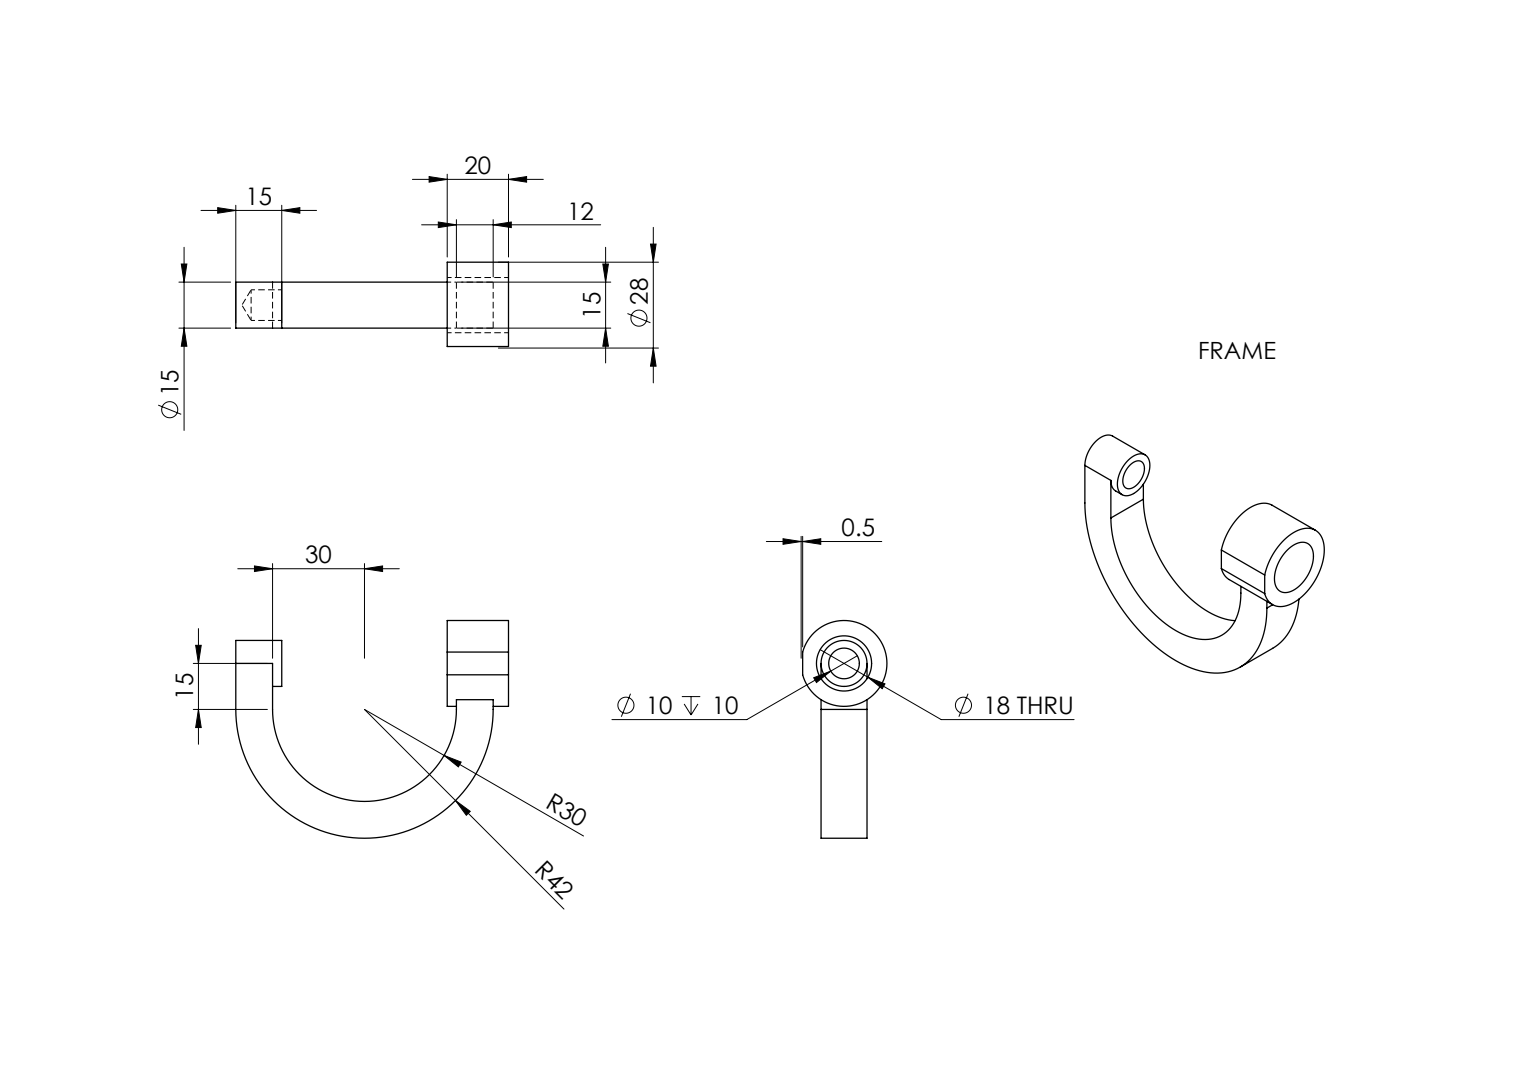
ISO-10303-21;
HEADER;
FILE_DESCRIPTION (('STEP AP214'),
    '1' );
FILE_NAME ('frame.step',
    '2026-10-22T12:35:56',
    ( '' ),
    ( '' ),
    'SwSTEP 2.0',
    'SolidWorks 2026',
    '' );
FILE_SCHEMA (( 'AUTOMOTIVE_DESIGN' ));
ENDSEC;

DATA;
#1=CARTESIAN_POINT ( 'NONE',  ( -30.00000000000000000, -8.316621552948000372E-15, 7.500000000000000000 ) ) ;
#2=ORIENTED_EDGE ( 'NONE', *, *, #1476, .F. ) ;
#4=DIRECTION ( 'NONE',  ( 0.000000000000000000, -1.000000000000000000, 0.000000000000000000 ) ) ;
#7=EDGE_CURVE ( 'NONE', #417, #1789, #1947, .T. ) ;
#12=VECTOR ( 'NONE', #2247, 1000.000000000000000 ) ;
#13=ORIENTED_EDGE ( 'NONE', *, *, #713, .T. ) ;
#15=CARTESIAN_POINT ( 'NONE',  ( 41.99999999999999289, -11.82159041753687845, 15.00000000000000000 ) ) ;
#16=CARTESIAN_POINT ( 'NONE',  ( 37.48326775981565362, -1.423407605072588344, 16.38680797912482134 ) ) ;
#23=CARTESIAN_POINT ( 'NONE',  ( -26.99999999999999645, -7.622732162557277534E-15, 7.500000000000000000 ) ) ;
#32=CIRCLE ( 'NONE', #2124, 4.999999999999998224 ) ;
#33=CARTESIAN_POINT ( 'NONE',  ( 30.00000000000000355, -15.00000000000000355, 15.00000000000000000 ) ) ;
#40=DIRECTION ( 'NONE',  ( 0.000000000000000000, 0.000000000000000000, -1.000000000000000000 ) ) ;
#47=DIRECTION ( 'NONE',  ( 0.5150380749100542666, 1.049727191138618572E-16, 0.8571673007021122226 ) ) ;
#51=EDGE_CURVE ( 'NONE', #357, #1877, #2331, .T. ) ;
#54=CARTESIAN_POINT ( 'NONE',  ( 35.50000000000001421, 0.09798730130381244630, 16.49999999999999645 ) ) ;
#56=VERTEX_POINT ( 'NONE', #623 ) ;
#57=ORIENTED_EDGE ( 'NONE', *, *, #1286, .T. ) ;
#60=DIRECTION ( 'NONE',  ( -2.478176394252581634E-16, 1.000000000000000000, 0.000000000000000000 ) ) ;
#63=COLOUR_RGB ( '',0.8941176470588234615, 0.8941176470588234615, 0.8941176470588234615 ) ;
#64=ORIENTED_EDGE ( 'NONE', *, *, #1192, .F. ) ;
#66=AXIS2_PLACEMENT_3D ( 'NONE', #1107, #1144, #2625 ) ;
#69=ORIENTED_EDGE ( 'NONE', *, *, #671, .F. ) ;
#71=CARTESIAN_POINT ( 'NONE',  ( 38.30162487582177278, 0.7519129166725618818, 16.46890859085320358 ) ) ;
#72=DIRECTION ( 'NONE',  ( -0.000000000000000000, -0.000000000000000000, 1.000000000000000000 ) ) ;
#73=CARTESIAN_POINT ( 'NONE',  ( 36.00776062886355078, -1.129166992945587866, 16.42915638304272363 ) ) ;
#76=EDGE_CURVE ( 'NONE', #916, #1503, #2106, .T. ) ;
#77=DIRECTION ( 'NONE',  ( 1.000000000000000000, 2.312964634635742957E-16, 0.000000000000000000 ) ) ;
#81=AXIS2_PLACEMENT_3D ( 'NONE', #778, #1048, #1778 ) ;
#86=DIRECTION ( 'NONE',  ( -2.312964634635742957E-16, 1.000000000000000000, 0.000000000000000000 ) ) ;
#87=VERTEX_POINT ( 'NONE', #874 ) ;
#96=ORIENTED_EDGE ( 'NONE', *, *, #1476, .T. ) ;
#97=ORIENTED_EDGE ( 'NONE', *, *, #671, .T. ) ;
#99=CARTESIAN_POINT ( 'NONE',  ( 37.00000000000000000, 1.474514954580286030E-14, 20.99999999999999645 ) ) ;
#102=AXIS2_PLACEMENT_3D ( 'NONE', #2450, #1198, #3216 ) ;
#107=CARTESIAN_POINT ( 'NONE',  ( 38.45998082922275785, -0.3957415549423216605, 16.49311123862704775 ) ) ;
#116=VECTOR ( 'NONE', #3173, 1000.000000000000000 ) ;
#118=DIRECTION ( 'NONE',  ( 0.000000000000000000, 0.000000000000000000, -1.000000000000000000 ) ) ;
#120=DIRECTION ( 'NONE',  ( 1.000000000000000000, 2.312964634635742957E-16, -0.000000000000000000 ) ) ;
#121=AXIS2_PLACEMENT_3D ( 'NONE', #2014, #774, #60 ) ;
#127=ADVANCED_FACE ( 'NONE', ( #378 ), #1155, .F. ) ;
#128=ADVANCED_FACE ( 'NONE', ( #911 ), #1859, .T. ) ;
#129=ORIENTED_EDGE ( 'NONE', *, *, #314, .F. ) ;
#134=CYLINDRICAL_SURFACE ( 'NONE', #2744, 14.00000000000000000 ) ;
#136=ORIENTED_EDGE ( 'NONE', *, *, #525, .F. ) ;
#147=EDGE_CURVE ( 'NONE', #1882, #2430, #639, .T. ) ;
#148=CYLINDRICAL_SURFACE ( 'NONE', #941, 7.500000000000000000 ) ;
#158=CARTESIAN_POINT ( 'NONE',  ( 41.99999999999999289, 6.449497959004948951E-15, 15.00000000000000000 ) ) ;
#163=VERTEX_POINT ( 'NONE', #411 ) ;
#167=DIRECTION ( 'NONE',  ( -0.000000000000000000, -0.000000000000000000, -1.000000000000000000 ) ) ;
#172=AXIS2_PLACEMENT_3D ( 'NONE', #834, #880, #1605 ) ;
#177=ORIENTED_EDGE ( 'NONE', *, *, #295, .F. ) ;
#190=DIRECTION ( 'NONE',  ( 1.000000000000000000, -0.000000000000000000, -0.000000000000000000 ) ) ;
#193=CIRCLE ( 'NONE', #2951, 14.00000000000000000 ) ;
#198=CYLINDRICAL_SURFACE ( 'NONE', #340, 1.499999999999994449 ) ;
#204=LINE ( 'NONE', #1443, #277 ) ;
#206=CONICAL_SURFACE ( 'NONE', #1038, 4.999999999999998224, 1.029744258676654312 ) ;
#210=ADVANCED_FACE ( 'NONE', ( #1707 ), #1221, .T. ) ;
#216=CARTESIAN_POINT ( 'NONE',  ( -41.99999999999999289, -6.449497959004950529E-15, 0.000000000000000000 ) ) ;
#217=DIRECTION ( 'NONE',  ( 0.000000000000000000, 0.000000000000000000, -1.000000000000000000 ) ) ;
#218=DIRECTION ( 'NONE',  ( 1.000000000000000000, 0.000000000000000000, 0.000000000000000000 ) ) ;
#224=AXIS2_PLACEMENT_3D ( 'NONE', #361, #2327, #86 ) ;
#226=AXIS2_PLACEMENT_3D ( 'NONE', #781, #362, #1550 ) ;
#227=DIRECTION ( 'NONE',  ( -1.000000000000000000, -2.312964634635742957E-16, 0.000000000000000000 ) ) ;
#231=ORIENTED_EDGE ( 'NONE', *, *, #2924, .F. ) ;
#232=EDGE_LOOP ( 'NONE', ( #1435, #2607, #784, #823 ) ) ;
#246=CIRCLE ( 'NONE', #2580, 14.00000000000000000 ) ;
#247=ORIENTED_EDGE ( 'NONE', *, *, #3182, .F. ) ;
#254=PRODUCT_DEFINITION ( 'UNKNOWN', '', #1654, #571 ) ;
#259=CARTESIAN_POINT ( 'NONE',  ( 27.00000000000000000, 6.704247063196759979E-15, 7.500000000000000000 ) ) ;
#266=DIRECTION ( 'NONE',  ( -2.478176394252581634E-16, 1.000000000000000000, 0.000000000000000000 ) ) ;
#273=EDGE_CURVE ( 'NONE', #3128, #417, #1689, .T. ) ;
#276=DIRECTION ( 'NONE',  ( 1.000000000000000000, 0.000000000000000000, 0.000000000000000000 ) ) ;
#277=VECTOR ( 'NONE', #2201, 1000.000000000000000 ) ;
#279=CARTESIAN_POINT ( 'NONE',  ( -41.99999999999999289, -1.109217911451089172E-14, 0.000000000000000000 ) ) ;
#282=CIRCLE ( 'NONE', #2213, 4.999999999999999112 ) ;
#287=CARTESIAN_POINT ( 'NONE',  ( 38.19805860116020568, -0.9234461779904078460, 16.45357685834587613 ) ) ;
#289=LINE ( 'NONE', #2050, #12 ) ;
#295=EDGE_CURVE ( 'NONE', #1128, #2739, #2239, .T. ) ;
#297=PLANE ( 'NONE',  #1247 ) ;
#299=ORIENTED_EDGE ( 'NONE', *, *, #397, .F. ) ;
#308=DIRECTION ( 'NONE',  ( -1.000000000000000000, -2.312964634635742957E-16, 0.000000000000000000 ) ) ;
#313=FACE_OUTER_BOUND ( 'NONE', #2374, .T. ) ;
#314=EDGE_CURVE ( 'NONE', #1882, #2739, #2737, .T. ) ;
#317=DIRECTION ( 'NONE',  ( -2.312964634635742957E-16, 1.000000000000000000, -0.000000000000000000 ) ) ;
#320=ORIENTED_EDGE ( 'NONE', *, *, #1335, .T. ) ;
#324=ORIENTED_EDGE ( 'NONE', *, *, #2185, .F. ) ;
#325=ADVANCED_FACE ( 'NONE', ( #447 ), #1432, .F. ) ;
#327=CARTESIAN_POINT ( 'NONE',  ( 38.49999999999999289, 1.474514954580286030E-14, 16.49999999999999289 ) ) ;
#329=EDGE_CURVE ( 'NONE', #2636, #2004, #2214, .T. ) ;
#333=CIRCLE ( 'NONE', #2770, 14.00000000000000000 ) ;
#335=CARTESIAN_POINT ( 'NONE',  ( -30.00000000000000000, -3.673940397442059178E-15, 0.000000000000000000 ) ) ;
#340=AXIS2_PLACEMENT_3D ( 'NONE', #664, #915, #276 ) ;
#341=AXIS2_PLACEMENT_3D ( 'NONE', #259, #1766, #1051 ) ;
#346=CYLINDRICAL_SURFACE ( 'NONE', #226, 14.00000000000000000 ) ;
#349=ORIENTED_EDGE ( 'NONE', *, *, #2340, .F. ) ;
#353=FACE_OUTER_BOUND ( 'NONE', #1646, .T. ) ;
#355=FACE_OUTER_BOUND ( 'NONE', #984, .T. ) ;
#357=VERTEX_POINT ( 'NONE', #15 ) ;
#361=CARTESIAN_POINT ( 'NONE',  ( 47.00000000000000000, 1.133017633246824530E-14, 7.500000000000000000 ) ) ;
#362=DIRECTION ( 'NONE',  ( 1.000000000000000000, 2.312964634635742957E-16, 0.000000000000000000 ) ) ;
#363=DIRECTION ( 'NONE',  ( -0.000000000000000000, -0.000000000000000000, -1.000000000000000000 ) ) ;
#366=CARTESIAN_POINT ( 'NONE',  ( 38.50000000000000000, -0.1985404316418107051, 16.49999999999999645 ) ) ;
#367=ORIENTED_EDGE ( 'NONE', *, *, #1335, .F. ) ;
#372=EDGE_CURVE ( 'NONE', #87, #2397, #1009, .T. ) ;
#378=FACE_OUTER_BOUND ( 'NONE', #1451, .T. ) ;
#382=ORIENTED_EDGE ( 'NONE', *, *, #1088, .F. ) ;
#386=AXIS2_PLACEMENT_3D ( 'NONE', #1799, #2316, #40 ) ;
#389=EDGE_LOOP ( 'NONE', ( #1124, #807, #247, #64 ) ) ;
#390=AXIS2_PLACEMENT_3D ( 'NONE', #3020, #1047, #980 ) ;
#392=VECTOR ( 'NONE', #317, 1000.000000000000000 ) ;
#393=DIRECTION ( 'NONE',  ( -1.000000000000000000, -2.312964634635742957E-16, 0.000000000000000000 ) ) ;
#397=EDGE_CURVE ( 'NONE', #1789, #2998, #1521, .T. ) ;
#410=VECTOR ( 'NONE', #420, 1000.000000000000000 ) ;
#411=CARTESIAN_POINT ( 'NONE',  ( 27.00000000000000000, 1.243235845170086479E-14, 16.49999999999999289 ) ) ;
#417=VERTEX_POINT ( 'NONE', #1239 ) ;
#420=DIRECTION ( 'NONE',  ( 1.000000000000000000, 2.312964634635742957E-16, 0.000000000000000000 ) ) ;
#424=VECTOR ( 'NONE', #2474, 1000.000000000000000 ) ;
#434=DIRECTION ( 'NONE',  ( -2.312964634635742957E-16, 1.000000000000000000, 0.000000000000000000 ) ) ;
#435=DIRECTION ( 'NONE',  ( 1.000000000000000000, 2.312964634635742957E-16, 0.000000000000000000 ) ) ;
#440=CARTESIAN_POINT ( 'NONE',  ( -41.99999999999999289, -15.00000000000000711, 15.00000000000000000 ) ) ;
#443=CLOSED_SHELL ( 'NONE', ( #3157, #127, #2028, #1449, #2628, #1324, #3219, #537, #1757, #1948, #128, #2460, #2730, #325, #210, #2684, #2552, #1070, #2797, #829, #2086, #2736, #3198, #1675, #3211 ) ) ;
#447=FACE_OUTER_BOUND ( 'NONE', #1253, .T. ) ;
#450=CYLINDRICAL_SURFACE ( 'NONE', #386, 8.999999999999994671 ) ;
#452=CARTESIAN_POINT ( 'NONE',  ( -26.99999999999999645, -7.622732162557277534E-15, 7.500000000000000000 ) ) ;
#464=ORIENTED_EDGE ( 'NONE', *, *, #1403, .T. ) ;
#469=DIRECTION ( 'NONE',  ( -0.000000000000000000, -0.000000000000000000, -1.000000000000000000 ) ) ;
#470=DIRECTION ( 'NONE',  ( 0.000000000000000000, 0.000000000000000000, -1.000000000000000000 ) ) ;
#485=PRODUCT_CONTEXT ( 'NONE', #2078, 'mechanical' ) ;
#491=( GEOMETRIC_REPRESENTATION_CONTEXT ( 3 ) GLOBAL_UNCERTAINTY_ASSIGNED_CONTEXT ( ( #2017 ) ) GLOBAL_UNIT_ASSIGNED_CONTEXT ( ( #605, #1315, #1563 ) ) REPRESENTATION_CONTEXT ( 'NONE', 'WORKASPACE' ) );
#505=FACE_BOUND ( 'NONE', #645, .T. ) ;
#508=CARTESIAN_POINT ( 'NONE',  ( 35.50982285435565444, 0.1975270956567308500, 16.49834805537327043 ) ) ;
#511=DIRECTION ( 'NONE',  ( 1.000000000000000000, 0.000000000000000000, 0.000000000000000000 ) ) ;
#514=SHAPE_REPRESENTATION ( 'frame', ( #2878 ), #491 ) ;
#515=CIRCLE ( 'NONE', #769, 14.00000000000000000 ) ;
#522=DIRECTION ( 'NONE',  ( -0.000000000000000000, -0.000000000000000000, 1.000000000000000000 ) ) ;
#525=EDGE_CURVE ( 'NONE', #974, #2998, #2583, .T. ) ;
#526=CARTESIAN_POINT ( 'NONE',  ( 37.92226537325436198, 1.198992358192679797, 16.42086068928975706 ) ) ;
#529=ORIENTED_EDGE ( 'NONE', *, *, #1753, .F. ) ;
#530=CIRCLE ( 'NONE', #1202, 8.999999999999989342 ) ;
#532=DIRECTION ( 'NONE',  ( 1.000000000000000000, 2.312964634635742957E-16, 0.000000000000000000 ) ) ;
#533=CARTESIAN_POINT ( 'NONE',  ( 37.99089481476345753, -1.130332597043731901, 16.42900728359812135 ) ) ;
#537=ADVANCED_FACE ( 'NONE', ( #579 ), #1568, .T. ) ;
#538=CARTESIAN_POINT ( 'NONE',  ( -26.99999999999999645, -7.622732162557277534E-15, 7.500000000000000000 ) ) ;
#542=SURFACE_STYLE_FILL_AREA ( #2023 ) ;
#553=CARTESIAN_POINT ( 'NONE',  ( 35.68903409116789760, -0.7546922429561464529, 16.47012649564899078 ) ) ;
#559=EDGE_CURVE ( 'NONE', #3128, #1393, #1428, .T. ) ;
#561=CARTESIAN_POINT ( 'NONE',  ( 35.50000000000000000, 1.243235838461289750E-14, 16.49999999999999289 ) ) ;
#564=ORIENTED_EDGE ( 'NONE', *, *, #1430, .T. ) ;
#571=PRODUCT_DEFINITION_CONTEXT ( 'detailed design', #2741, 'design' ) ;
#574=DIRECTION ( 'NONE',  ( 1.000000000000000000, 0.000000000000000000, 0.000000000000000000 ) ) ;
#575=EDGE_CURVE ( 'NONE', #2092, #576, #3015, .T. ) ;
#576=VERTEX_POINT ( 'NONE', #1290 ) ;
#579=FACE_OUTER_BOUND ( 'NONE', #389, .T. ) ;
#585=VERTEX_POINT ( 'NONE', #1541 ) ;
#586=CARTESIAN_POINT ( 'NONE',  ( -26.99999999999999645, -5.173438564262573782E-15, 12.49999999999999822 ) ) ;
#593=CARTESIAN_POINT ( 'NONE',  ( -30.00000000000000000, -3.673940397442059178E-15, 0.000000000000000000 ) ) ;
#596=ORIENTED_EDGE ( 'NONE', *, *, #1551, .F. ) ;
#598=EDGE_CURVE ( 'NONE', #1829, #1709, #1645, .T. ) ;
#599=VECTOR ( 'NONE', #47, 1000.000000000000000 ) ;
#600=AXIS2_PLACEMENT_3D ( 'NONE', #3063, #77, #3053 ) ;
#605=( LENGTH_UNIT ( ) NAMED_UNIT ( * ) SI_UNIT ( .MILLI., .METRE. ) );
#612=CARTESIAN_POINT ( 'NONE',  ( -26.99999999999999645, -5.785761963836251101E-15, 2.500000000000000444 ) ) ;
#613=AXIS2_PLACEMENT_3D ( 'NONE', #951, #1199, #470 ) ;
#623=CARTESIAN_POINT ( 'NONE',  ( -40.00430309513780003, -9.040569623688697978E-15, 7.500000000000000000 ) ) ;
#629=DIRECTION ( 'NONE',  ( -2.312964634635742957E-16, 1.000000000000000000, 0.000000000000000000 ) ) ;
#631=DIRECTION ( 'NONE',  ( -0.000000000000000000, -0.000000000000000000, -1.000000000000000000 ) ) ;
#639=LINE ( 'NONE', #1636, #1796 ) ;
#640=VERTEX_POINT ( 'NONE', #1514 ) ;
#645=EDGE_LOOP ( 'NONE', ( #2403, #3181 ) ) ;
#647=AXIS2_PLACEMENT_3D ( 'NONE', #686, #2975, #2223 ) ;
#650=CIRCLE ( 'NONE', #1368, 8.999999999999994671 ) ;
#654=AXIS2_PLACEMENT_3D ( 'NONE', #452, #2165, #917 ) ;
#657=EDGE_CURVE ( 'NONE', #1365, #640, #2412, .T. ) ;
#659=DIRECTION ( 'NONE',  ( 0.000000000000000000, 0.000000000000000000, -1.000000000000000000 ) ) ;
#662=DIRECTION ( 'NONE',  ( 1.000000000000000000, 2.312964634635742957E-16, 0.000000000000000000 ) ) ;
#664=CARTESIAN_POINT ( 'NONE',  ( 37.00000000000000000, 1.474514954580286030E-14, 20.99999999999999645 ) ) ;
#668=LINE ( 'NONE', #730, #1764 ) ;
#671=EDGE_CURVE ( 'NONE', #1489, #1964, #2710, .T. ) ;
#673=VECTOR ( 'NONE', #1742, 1000.000000000000000 ) ;
#682=CARTESIAN_POINT ( 'NONE',  ( 30.00000000000000355, -11.82159041753688200, 15.00000000000000000 ) ) ;
#686=CARTESIAN_POINT ( 'NONE',  ( 3.469446951953614189E-15, -15.00000000000000355, 15.00000000000000000 ) ) ;
#687=ORIENTED_EDGE ( 'NONE', *, *, #1176, .F. ) ;
#690=EDGE_LOOP ( 'NONE', ( #13, #3111, #3143, #1378, #349, #2589 ) ) ;
#693=CARTESIAN_POINT ( 'NONE',  ( -37.00000000000000000, -5.785761963836251101E-15, 2.500000000000001332 ) ) ;
#695=CARTESIAN_POINT ( 'NONE',  ( -29.99999999999999645, -15.00000000000000355, 15.00000000000000000 ) ) ;
#698=FACE_OUTER_BOUND ( 'NONE', #2603, .T. ) ;
#702=VECTOR ( 'NONE', #227, 1000.000000000000000 ) ;
#710=DIRECTION ( 'NONE',  ( 1.000000000000000000, -0.000000000000000000, -0.000000000000000000 ) ) ;
#713=EDGE_CURVE ( 'NONE', #1393, #3128, #2675, .T. ) ;
#727=DIRECTION ( 'NONE',  ( 0.000000000000000000, 1.000000000000000000, 0.000000000000000000 ) ) ;
#729=FACE_OUTER_BOUND ( 'NONE', #989, .T. ) ;
#730=CARTESIAN_POINT ( 'NONE',  ( 30.00000000000000355, -15.00000000000000355, 15.00000000000000000 ) ) ;
#732=DIRECTION ( 'NONE',  ( 1.000000000000000000, 2.312964634635742957E-16, 0.000000000000000000 ) ) ;
#736=CARTESIAN_POINT ( 'NONE',  ( 41.99999999999999289, -11.82159041753688022, 0.000000000000000000 ) ) ;
#741=FACE_OUTER_BOUND ( 'NONE', #2868, .T. ) ;
#746=VECTOR ( 'NONE', #732, 1000.000000000000000 ) ;
#750=DIRECTION ( 'NONE',  ( -0.000000000000000000, -0.000000000000000000, -1.000000000000000000 ) ) ;
#756=CARTESIAN_POINT ( 'NONE',  ( -37.00000000000000000, -5.173438564262574571E-15, 12.49999999999999645 ) ) ;
#762=DIRECTION ( 'NONE',  ( 1.000000000000000000, 0.000000000000000000, 0.000000000000000000 ) ) ;
#769=AXIS2_PLACEMENT_3D ( 'NONE', #3204, #435, #2416 ) ;
#772=EDGE_CURVE ( 'NONE', #1678, #1779, #333, .T. ) ;
#774=DIRECTION ( 'NONE',  ( 1.000000000000000000, 2.312964634635742957E-16, -0.000000000000000000 ) ) ;
#776=( LENGTH_UNIT ( ) NAMED_UNIT ( * ) SI_UNIT ( .MILLI., .METRE. ) );
#777=UNCERTAINTY_MEASURE_WITH_UNIT (LENGTH_MEASURE( 1.000000000000000082E-05 ), #1533, 'distance_accuracy_value', 'NONE');
#778=CARTESIAN_POINT ( 'NONE',  ( -41.99999999999999289, -1.109217911451089172E-14, 7.500000000000000000 ) ) ;
#779=VERTEX_POINT ( 'NONE', #586 ) ;
#781=CARTESIAN_POINT ( 'NONE',  ( 27.00000000000000000, 6.704247063196759979E-15, 7.500000000000000000 ) ) ;
#782=CARTESIAN_POINT ( 'NONE',  ( -26.99999999999999645, -5.785761963836251101E-15, 7.500000000000000000 ) ) ;
#784=ORIENTED_EDGE ( 'NONE', *, *, #2418, .T. ) ;
#790=AXIS2_PLACEMENT_3D ( 'NONE', #2216, #1953, #2198 ) ;
#792=LINE ( 'NONE', #2780, #2329 ) ;
#796=CARTESIAN_POINT ( 'NONE',  ( 35.54829862735515889, 0.3901384415568778796, 16.49205630963118807 ) ) ;
#801=( GEOMETRIC_REPRESENTATION_CONTEXT ( 3 ) GLOBAL_UNCERTAINTY_ASSIGNED_CONTEXT ( ( #1879 ) ) GLOBAL_UNIT_ASSIGNED_CONTEXT ( ( #776, #1509, #3040 ) ) REPRESENTATION_CONTEXT ( 'NONE', 'WORKASPACE' ) );
#802=ORIENTED_EDGE ( 'NONE', *, *, #575, .T. ) ;
#804=DIRECTION ( 'NONE',  ( 0.000000000000000000, -1.000000000000000000, 0.000000000000000000 ) ) ;
#807=ORIENTED_EDGE ( 'NONE', *, *, #1490, .T. ) ;
#818=LINE ( 'NONE', #756, #599 ) ;
#823=ORIENTED_EDGE ( 'NONE', *, *, #2248, .T. ) ;
#825=CARTESIAN_POINT ( 'NONE',  ( 35.80758137781341333, 0.9152444266664423456, 16.45371270176149991 ) ) ;
#826=FILL_AREA_STYLE_COLOUR ( '', #63 ) ;
#829=ADVANCED_FACE ( 'NONE', ( #1330, #2376 ), #1614, .T. ) ;
#833=ORIENTED_EDGE ( 'NONE', *, *, #2536, .F. ) ;
#834=CARTESIAN_POINT ( 'NONE',  ( 27.00000000000000000, 1.133017633246824530E-14, 7.500000000000000000 ) ) ;
#835=DIRECTION ( 'NONE',  ( 1.000000000000000000, 2.312964634635742957E-16, 0.000000000000000000 ) ) ;
#837=DIRECTION ( 'NONE',  ( -0.000000000000000000, -0.000000000000000000, -1.000000000000000000 ) ) ;
#839=EDGE_CURVE ( 'NONE', #1877, #916, #3032, .T. ) ;
#840=ORIENTED_EDGE ( 'NONE', *, *, #1067, .T. ) ;
#846=CARTESIAN_POINT ( 'NONE',  ( -29.99999999999999645, -15.00000000000000355, 15.00000000000000000 ) ) ;
#859=ORIENTED_EDGE ( 'NONE', *, *, #1403, .F. ) ;
#864=CIRCLE ( 'NONE', #81, 7.500000000000000000 ) ;
#869=VECTOR ( 'NONE', #662, 1000.000000000000000 ) ;
#871=FACE_OUTER_BOUND ( 'NONE', #3146, .T. ) ;
#874=CARTESIAN_POINT ( 'NONE',  ( 47.00000000000000000, -13.99999999999998757, 7.500000000000001776 ) ) ;
#877=VERTEX_POINT ( 'NONE', #2663 ) ;
#880=DIRECTION ( 'NONE',  ( 1.000000000000000000, 2.312964634635742957E-16, 0.000000000000000000 ) ) ;
#883=CARTESIAN_POINT ( 'NONE',  ( 47.00000000000000000, 1.133017633246824530E-14, 7.500000000000000000 ) ) ;
#893=EDGE_CURVE ( 'NONE', #2713, #2821, #204, .T. ) ;
#895=ORIENTED_EDGE ( 'NONE', *, *, #314, .T. ) ;
#900=AXIS2_PLACEMENT_3D ( 'NONE', #2362, #363, #3105 ) ;
#907=PRODUCT_DEFINITION_SHAPE ( 'NONE', 'NONE',  #254 ) ;
#911=FACE_OUTER_BOUND ( 'NONE', #2074, .T. ) ;
#915=DIRECTION ( 'NONE',  ( -0.000000000000000000, -0.000000000000000000, 1.000000000000000000 ) ) ;
#916=VERTEX_POINT ( 'NONE', #440 ) ;
#917=DIRECTION ( 'NONE',  ( 0.000000000000000000, -1.000000000000000000, 0.000000000000000000 ) ) ;
#918=CARTESIAN_POINT ( 'NONE',  ( -26.99999999999999645, -5.785761963836251101E-15, 7.500000000000000000 ) ) ;
#924=CARTESIAN_POINT ( 'NONE',  ( 27.00000000000000355, -11.82159041753688200, 15.00000000000000000 ) ) ;
#930=CARTESIAN_POINT ( 'NONE',  ( 52.00000000000000711, 3.708099243547853252, 20.99999999999999645 ) ) ;
#931=EDGE_CURVE ( 'NONE', #1570, #585, #2261, .T. ) ;
#933=ORIENTED_EDGE ( 'NONE', *, *, #2759, .F. ) ;
#941=AXIS2_PLACEMENT_3D ( 'NONE', #1146, #2146, #3131 ) ;
#943=EDGE_CURVE ( 'NONE', #2713, #357, #3155, .T. ) ;
#951=CARTESIAN_POINT ( 'NONE',  ( -37.00000000000000000, -5.785761963836251101E-15, 7.500000000000000000 ) ) ;
#960=PLANE ( 'NONE',  #1825 ) ;
#962=ORIENTED_EDGE ( 'NONE', *, *, #893, .T. ) ;
#966=FACE_OUTER_BOUND ( 'NONE', #1512, .T. ) ;
#973=CARTESIAN_POINT ( 'NONE',  ( 41.99999999999999289, -15.00000000000000355, 15.00000000000000000 ) ) ;
#974=VERTEX_POINT ( 'NONE', #1187 ) ;
#978=CARTESIAN_POINT ( 'NONE',  ( -30.00000000000000000, -7.500000000000007994, 7.500000000000000000 ) ) ;
#980=DIRECTION ( 'NONE',  ( 0.000000000000000000, 0.000000000000000000, -1.000000000000000000 ) ) ;
#984=EDGE_LOOP ( 'NONE', ( #2241, #2447, #2019, #1978, #3024, #2576, #596, #895 ) ) ;
#989=EDGE_LOOP ( 'NONE', ( #2526, #57, #564, #96, #3116, #3195, #136, #1328 ) ) ;
#992=CARTESIAN_POINT ( 'NONE',  ( 36.60604563826976943, -1.460666791800804498, 16.38100777177576362 ) ) ;
#1002=CARTESIAN_POINT ( 'NONE',  ( 35.86950496355626683, 0.9908260551213666778, 16.44556929574713777 ) ) ;
#1005=DIRECTION ( 'NONE',  ( -0.000000000000000000, -0.000000000000000000, 1.000000000000000000 ) ) ;
#1007=LINE ( 'NONE', #2488, #424 ) ;
#1009=CIRCLE ( 'NONE', #2315, 14.00000000000000000 ) ;
#1012=ORIENTED_EDGE ( 'NONE', *, *, #772, .T. ) ;
#1021=AXIS2_PLACEMENT_3D ( 'NONE', #1457, #2451, #218 ) ;
#1031=CONICAL_SURFACE ( 'NONE', #613, 4.999999999999998224, 1.029744258676654312 ) ;
#1033=ORIENTED_EDGE ( 'NONE', *, *, #2418, .F. ) ;
#1036=PRESENTATION_STYLE_ASSIGNMENT (( #1283 ) ) ;
#1038=AXIS2_PLACEMENT_3D ( 'NONE', #2152, #1475, #2436 ) ;
#1040=CARTESIAN_POINT ( 'NONE',  ( -26.99999999999999645, -7.622732162557277534E-15, 7.500000000000000000 ) ) ;
#1041=CARTESIAN_POINT ( 'NONE',  ( 36.08479696852054985, -1.192462354422064497, 16.42082098627955844 ) ) ;
#1046=AXIS2_PLACEMENT_3D ( 'NONE', #2529, #2745, #266 ) ;
#1047=DIRECTION ( 'NONE',  ( 1.000000000000000000, -0.000000000000000000, -0.000000000000000000 ) ) ;
#1048=DIRECTION ( 'NONE',  ( -1.000000000000000000, -2.312964634635742957E-16, 0.000000000000000000 ) ) ;
#1050=ADVANCED_BREP_SHAPE_REPRESENTATION ( '', ( #2136, #2878 ), #491 ) ;
#1051=DIRECTION ( 'NONE',  ( -2.478176394252581634E-16, 1.000000000000000000, 0.000000000000000000 ) ) ;
#1052=FACE_OUTER_BOUND ( 'NONE', #1325, .T. ) ;
#1055=DIRECTION ( 'NONE',  ( -1.000000000000000000, -2.312964634635742957E-16, 0.000000000000000000 ) ) ;
#1056=ORIENTED_EDGE ( 'NONE', *, *, #1551, .T. ) ;
#1058=ORIENTED_EDGE ( 'NONE', *, *, #76, .F. ) ;
#1060=AXIS2_PLACEMENT_3D ( 'NONE', #1040, #1830, #804 ) ;
#1067=EDGE_CURVE ( 'NONE', #2004, #2636, #3079, .T. ) ;
#1068=DIRECTION ( 'NONE',  ( 0.000000000000000000, 1.000000000000000000, 0.000000000000000000 ) ) ;
#1069=ORIENTED_EDGE ( 'NONE', *, *, #1430, .F. ) ;
#1070=ADVANCED_FACE ( 'NONE', ( #505, #1762 ), #1495, .F. ) ;
#1071=CARTESIAN_POINT ( 'NONE',  ( 36.80294994545206322, 1.490236770648136089, 16.37578575999040353 ) ) ;
#1072=ORIENTED_EDGE ( 'NONE', *, *, #7, .T. ) ;
#1077=LINE ( 'NONE', #612, #2159 ) ;
#1079=EDGE_LOOP ( 'NONE', ( #933, #177, #3058, #1169 ) ) ;
#1080=EDGE_CURVE ( 'NONE', #2998, #1599, #2718, .T. ) ;
#1082=( NAMED_UNIT ( * ) PLANE_ANGLE_UNIT ( ) SI_UNIT ( $, .RADIAN. ) );
#1087=CARTESIAN_POINT ( 'NONE',  ( 30.00000000000000000, 3.673940397442057600E-15, 0.000000000000000000 ) ) ;
#1088=EDGE_CURVE ( 'NONE', #1709, #1829, #32, .T. ) ;
#1092=EDGE_CURVE ( 'NONE', #3031, #417, #864, .T. ) ;
#1097=DIRECTION ( 'NONE',  ( 1.000000000000000000, 0.000000000000000000, 0.000000000000000000 ) ) ;
#1105=VECTOR ( 'NONE', #1744, 1000.000000000000000 ) ;
#1106=ORIENTED_EDGE ( 'NONE', *, *, #1172, .F. ) ;
#1107=CARTESIAN_POINT ( 'NONE',  ( 3.469446951953614189E-15, -15.00000000000000355, 15.00000000000000000 ) ) ;
#1110=CARTESIAN_POINT ( 'NONE',  ( 47.00000000000000000, 14.00000000000001243, 7.500000000000000000 ) ) ;
#1124=ORIENTED_EDGE ( 'NONE', *, *, #1408, .F. ) ;
#1127=EDGE_CURVE ( 'NONE', #3031, #1482, #792, .T. ) ;
#1128=VERTEX_POINT ( 'NONE', #2544 ) ;
#1132=VECTOR ( 'NONE', #1607, 1000.000000000000000 ) ;
#1133=CARTESIAN_POINT ( 'NONE',  ( 27.00000000000000000, 6.704247063196759979E-15, 7.500000000000000000 ) ) ;
#1134=VERTEX_POINT ( 'NONE', #2295 ) ;
#1141=ORIENTED_EDGE ( 'NONE', *, *, #76, .T. ) ;
#1144=DIRECTION ( 'NONE',  ( -0.000000000000000000, -0.000000000000000000, -1.000000000000000000 ) ) ;
#1146=CARTESIAN_POINT ( 'NONE',  ( -26.99999999999999645, -7.622732162557277534E-15, 7.500000000000000000 ) ) ;
#1148=CARTESIAN_POINT ( 'NONE',  ( 27.00000000000000355, -13.99999999999999467, 7.500000000000001776 ) ) ;
#1155=CYLINDRICAL_SURFACE ( 'NONE', #1262, 8.999999999999994671 ) ;
#1165=CARTESIAN_POINT ( 'NONE',  ( 26.99999999999999645, 14.00000000000000711, 7.500000000000000000 ) ) ;
#1169=ORIENTED_EDGE ( 'NONE', *, *, #657, .F. ) ;
#1171=DIRECTION ( 'NONE',  ( 0.000000000000000000, 0.000000000000000000, -1.000000000000000000 ) ) ;
#1172=EDGE_CURVE ( 'NONE', #1877, #877, #3057, .T. ) ;
#1176=EDGE_CURVE ( 'NONE', #1134, #1570, #1853, .T. ) ;
#1187=CARTESIAN_POINT ( 'NONE',  ( -29.99999999999999645, -15.00000000000000355, 0.000000000000000000 ) ) ;
#1192=EDGE_CURVE ( 'NONE', #2397, #2430, #193, .T. ) ;
#1195=DIRECTION ( 'NONE',  ( -1.000000000000000000, -2.312964634635743450E-16, -0.000000000000000000 ) ) ;
#1198=DIRECTION ( 'NONE',  ( 1.000000000000000000, 2.312964634635742957E-16, 0.000000000000000000 ) ) ;
#1199=DIRECTION ( 'NONE',  ( 1.000000000000000000, -0.000000000000000000, -0.000000000000000000 ) ) ;
#1201=CARTESIAN_POINT ( 'NONE',  ( 47.00000000000000000, 1.133017633246824530E-14, 7.500000000000000000 ) ) ;
#1202=AXIS2_PLACEMENT_3D ( 'NONE', #1630, #2958, #1171 ) ;
#1212=CARTESIAN_POINT ( 'NONE',  ( -30.00000000000000000, -8.316621552948000372E-15, 15.00000000000000000 ) ) ;
#1221=PLANE ( 'NONE',  #647 ) ;
#1225=ORIENTED_EDGE ( 'NONE', *, *, #2062, .T. ) ;
#1229=LINE ( 'NONE', #2968, #1309 ) ;
#1233=VECTOR ( 'NONE', #2894, 1000.000000000000000 ) ;
#1236=CARTESIAN_POINT ( 'NONE',  ( 3.469446951953614189E-15, -15.00000000000000355, 0.000000000000000000 ) ) ;
#1237=ORIENTED_EDGE ( 'NONE', *, *, #295, .T. ) ;
#1239=CARTESIAN_POINT ( 'NONE',  ( -41.99999999999999289, 7.499999999999988454, 7.500000000000000888 ) ) ;
#1247=AXIS2_PLACEMENT_3D ( 'NONE', #3011, #1055, #2024 ) ;
#1248=CARTESIAN_POINT ( 'NONE',  ( 38.12949724085409997, 0.9918543271721460552, 16.44544909559322932 ) ) ;
#1249=CARTESIAN_POINT ( 'NONE',  ( -26.99999999999999645, 7.499999999999992006, 7.500000000000000888 ) ) ;
#1253=EDGE_LOOP ( 'NONE', ( #1918, #1934, #2174, #320 ) ) ;
#1254=DIRECTION ( 'NONE',  ( 1.000000000000000000, 2.312964634635743450E-16, 0.000000000000000000 ) ) ;
#1255=CARTESIAN_POINT ( 'NONE',  ( 36.80088933932602657, -1.499879510127380522, 16.37414004115126431 ) ) ;
#1258=AXIS2_PLACEMENT_3D ( 'NONE', #2990, #522, #762 ) ;
#1260=CARTESIAN_POINT ( 'NONE',  ( -37.00000000000000000, -5.785761963836251101E-15, 7.500000000000000000 ) ) ;
#1262=AXIS2_PLACEMENT_3D ( 'NONE', #2618, #2901, #659 ) ;
#1271=AXIS2_PLACEMENT_3D ( 'NONE', #23, #2252, #4 ) ;
#1277=CARTESIAN_POINT ( 'NONE',  ( -26.99999999999999645, -5.785761963836251101E-15, 7.500000000000000000 ) ) ;
#1280=ORIENTED_EDGE ( 'NONE', *, *, #329, .F. ) ;
#1283=SURFACE_STYLE_USAGE ( .BOTH. , #1597 ) ;
#1286=EDGE_CURVE ( 'NONE', #2092, #1779, #1374, .T. ) ;
#1290=CARTESIAN_POINT ( 'NONE',  ( 30.00000000000000355, -15.00000000000000355, 0.000000000000000000 ) ) ;
#1292=CARTESIAN_POINT ( 'NONE',  ( -26.99999999999999645, -5.173438564262573782E-15, 12.49999999999999822 ) ) ;
#1293=EDGE_LOOP ( 'NONE', ( #2363, #69, #2551, #840 ) ) ;
#1294=DIRECTION ( 'NONE',  ( 0.000000000000000000, 0.000000000000000000, -1.000000000000000000 ) ) ;
#1295=DIRECTION ( 'NONE',  ( 1.000000000000000000, 2.312964634635743450E-16, 0.000000000000000000 ) ) ;
#1303=EDGE_CURVE ( 'NONE', #2965, #1482, #1593, .T. ) ;
#1309=VECTOR ( 'NONE', #1439, 1000.000000000000000 ) ;
#1314=CARTESIAN_POINT ( 'NONE',  ( 37.39427925860091051, 1.460378464396937304, 16.38104908776753277 ) ) ;
#1315=( NAMED_UNIT ( * ) PLANE_ANGLE_UNIT ( ) SI_UNIT ( $, .RADIAN. ) );
#1324=ADVANCED_FACE ( 'NONE', ( #355 ), #134, .T. ) ;
#1325=EDGE_LOOP ( 'NONE', ( #859, #2531, #1528, #2705, #1558, #97 ) ) ;
#1326=DIRECTION ( 'NONE',  ( -1.000000000000000000, -2.312964634635742957E-16, 0.000000000000000000 ) ) ;
#1328=ORIENTED_EDGE ( 'NONE', *, *, #1821, .F. ) ;
#1330=FACE_OUTER_BOUND ( 'NONE', #2812, .T. ) ;
#1335=EDGE_CURVE ( 'NONE', #2821, #576, #668, .T. ) ;
#1343=ORIENTED_EDGE ( 'NONE', *, *, #1408, .T. ) ;
#1348=DIRECTION ( 'NONE',  ( -2.312964634635742957E-16, 1.000000000000000000, 0.000000000000000000 ) ) ;
#1351=CARTESIAN_POINT ( 'NONE',  ( 38.49999999999999289, 1.474514954580286030E-14, 16.49999999999999289 ) ) ;
#1357=ORIENTED_EDGE ( 'NONE', *, *, #2924, .T. ) ;
#1358=ORIENTED_EDGE ( 'NONE', *, *, #1080, .T. ) ;
#1359=DIRECTION ( 'NONE',  ( -2.312964634635742957E-16, 1.000000000000000000, 0.000000000000000000 ) ) ;
#1360=CARTESIAN_POINT ( 'NONE',  ( 41.99999999999999289, 1.017369401515037180E-14, 7.500000000000000000 ) ) ;
#1365=VERTEX_POINT ( 'NONE', #1148 ) ;
#1368=AXIS2_PLACEMENT_3D ( 'NONE', #1909, #2016, #2777 ) ;
#1374=LINE ( 'NONE', #2067, #2691 ) ;
#1378=ORIENTED_EDGE ( 'NONE', *, *, #1127, .T. ) ;
#1379=CARTESIAN_POINT ( 'NONE',  ( 35.50000000000000000, 1.243235838461289750E-14, 16.49999999999999289 ) ) ;
#1389=ORIENTED_EDGE ( 'NONE', *, *, #2656, .F. ) ;
#1393=VERTEX_POINT ( 'NONE', #2927 ) ;
#1401=LINE ( 'NONE', #3147, #2161 ) ;
#1403=EDGE_CURVE ( 'NONE', #163, #1964, #2183, .T. ) ;
#1405=CIRCLE ( 'NONE', #2651, 30.00000000000000000 ) ;
#1408=EDGE_CURVE ( 'NONE', #640, #2397, #2167, .T. ) ;
#1410=STYLED_ITEM('',(#3236),#2136);
#1411=ORIENTED_EDGE ( 'NONE', *, *, #1303, .F. ) ;
#1428=CIRCLE ( 'NONE', #1060, 7.500000000000000000 ) ;
#1430=EDGE_CURVE ( 'NONE', #1779, #877, #1715, .T. ) ;
#1432=CYLINDRICAL_SURFACE ( 'NONE', #2465, 30.00000000000000000 ) ;
#1434=DIRECTION ( 'NONE',  ( -1.000000000000000000, 0.000000000000000000, -0.000000000000000000 ) ) ;
#1435=ORIENTED_EDGE ( 'NONE', *, *, #1508, .F. ) ;
#1436=LINE ( 'NONE', #1693, #2002 ) ;
#1439=DIRECTION ( 'NONE',  ( -2.312964634635742957E-16, 1.000000000000000000, 0.000000000000000000 ) ) ;
#1440=CARTESIAN_POINT ( 'NONE',  ( 47.00000000000000000, 1.243235845170086321E-14, 16.49999999999999289 ) ) ;
#1443=CARTESIAN_POINT ( 'NONE',  ( 30.00000000000000000, 3.673940397442057600E-15, 15.00000000000000000 ) ) ;
#1449=ADVANCED_FACE ( 'NONE', ( #966 ), #1031, .F. ) ;
#1451=EDGE_LOOP ( 'NONE', ( #2053, #464, #1357, #2567, #2755, #687 ) ) ;
#1457=CARTESIAN_POINT ( 'NONE',  ( 3.469446951953614189E-15, -15.00000000000000355, 0.000000000000000000 ) ) ;
#1467=EDGE_LOOP ( 'NONE', ( #3062, #1889 ) ) ;
#1469=CARTESIAN_POINT ( 'NONE',  ( 41.99999999999999289, 1.017369401515037180E-14, 7.500000000000000000 ) ) ;
#1471=FACE_OUTER_BOUND ( 'NONE', #1079, .T. ) ;
#1475=DIRECTION ( 'NONE',  ( 1.000000000000000000, -0.000000000000000000, -0.000000000000000000 ) ) ;
#1476=EDGE_CURVE ( 'NONE', #877, #1503, #2429, .T. ) ;
#1481=AXIS2_PLACEMENT_3D ( 'NONE', #3076, #1846, #2772 ) ;
#1482=VERTEX_POINT ( 'NONE', #1212 ) ;
#1489=VERTEX_POINT ( 'NONE', #2957 ) ;
#1490=EDGE_CURVE ( 'NONE', #640, #1128, #515, .T. ) ;
#1494=DIRECTION ( 'NONE',  ( 1.000000000000000000, -0.000000000000000000, -0.000000000000000000 ) ) ;
#1495=PLANE ( 'NONE',  #2507 ) ;
#1497=ORIENTED_EDGE ( 'NONE', *, *, #2340, .T. ) ;
#1503=VERTEX_POINT ( 'NONE', #1729 ) ;
#1508=EDGE_CURVE ( 'NONE', #1709, #779, #1543, .T. ) ;
#1509=( NAMED_UNIT ( * ) PLANE_ANGLE_UNIT ( ) SI_UNIT ( $, .RADIAN. ) );
#1511=DIRECTION ( 'NONE',  ( -1.000000000000000000, -2.312964634635742957E-16, 0.000000000000000000 ) ) ;
#1512=EDGE_LOOP ( 'NONE', ( #833, #1770, #1669 ) ) ;
#1514=CARTESIAN_POINT ( 'NONE',  ( 26.99999999999999645, 14.00000000000000711, 7.500000000000000000 ) ) ;
#1521=LINE ( 'NONE', #216, #3141 ) ;
#1528=ORIENTED_EDGE ( 'NONE', *, *, #1176, .T. ) ;
#1532=CARTESIAN_POINT ( 'NONE',  ( 36.51683924005257609, 1.423460261948054750, 16.38679996801885252 ) ) ;
#1533=( LENGTH_UNIT ( ) NAMED_UNIT ( * ) SI_UNIT ( .MILLI., .METRE. ) );
#1534=DIRECTION ( 'NONE',  ( 1.000000000000000000, -0.000000000000000000, -0.000000000000000000 ) ) ;
#1538=ORIENTED_EDGE ( 'NONE', *, *, #839, .F. ) ;
#1541=CARTESIAN_POINT ( 'NONE',  ( 47.00000000000000000, 1.243235845170086321E-14, 16.49999999999998579 ) ) ;
#1542=CARTESIAN_POINT ( 'NONE',  ( 36.24736826332972583, -1.301195037071565030, 16.40561087244777738 ) ) ;
#1543=LINE ( 'NONE', #1292, #673 ) ;
#1548=ORIENTED_EDGE ( 'NONE', *, *, #2033, .F. ) ;
#1549=CARTESIAN_POINT ( 'NONE',  ( 38.19275052663392245, 0.9148478194932688767, 16.45375607287287423 ) ) ;
#1550=DIRECTION ( 'NONE',  ( -2.478176394252581634E-16, 1.000000000000000000, 0.000000000000000000 ) ) ;
#1551=EDGE_CURVE ( 'NONE', #1882, #87, #246, .T. ) ;
#1554=ORIENTED_EDGE ( 'NONE', *, *, #329, .T. ) ;
#1558=ORIENTED_EDGE ( 'NONE', *, *, #3166, .F. ) ;
#1560=DIRECTION ( 'NONE',  ( 0.000000000000000000, -1.000000000000000000, 0.000000000000000000 ) ) ;
#1561=VERTEX_POINT ( 'NONE', #3017 ) ;
#1563=( NAMED_UNIT ( * ) SI_UNIT ( $, .STERADIAN. ) SOLID_ANGLE_UNIT ( ) );
#1567=ORIENTED_EDGE ( 'NONE', *, *, #1127, .F. ) ;
#1568=CYLINDRICAL_SURFACE ( 'NONE', #600, 14.00000000000000000 ) ;
#1570=VERTEX_POINT ( 'NONE', #1997 ) ;
#1572=CARTESIAN_POINT ( 'NONE',  ( -30.00000000000000000, -8.316621552948000372E-15, 7.500000000000000000 ) ) ;
#1593=LINE ( 'NONE', #2323, #3059 ) ;
#1597=SURFACE_SIDE_STYLE ('',( #542 ) ) ;
#1599=VERTEX_POINT ( 'NONE', #978 ) ;
#1602=AXIS2_PLACEMENT_3D ( 'NONE', #930, #2381, #1434 ) ;
#1605=DIRECTION ( 'NONE',  ( -3.854941057726240069E-16, 1.000000000000000000, 0.000000000000000000 ) ) ;
#1607=DIRECTION ( 'NONE',  ( 1.000000000000000000, -0.000000000000000000, -0.000000000000000000 ) ) ;
#1614=PLANE ( 'NONE',  #224 ) ;
#1624=CARTESIAN_POINT ( 'NONE',  ( 47.00000000000000000, 3.708099243547851920, 20.99999999999999645 ) ) ;
#1627=CIRCLE ( 'NONE', #1046, 14.00000000000000000 ) ;
#1629=EDGE_LOOP ( 'NONE', ( #231, #1908, #1554, #1673 ) ) ;
#1630=CARTESIAN_POINT ( 'NONE',  ( 47.00000000000000000, 1.133017633246824530E-14, 7.500000000000000000 ) ) ;
#1631=DIRECTION ( 'NONE',  ( 0.000000000000000000, 1.000000000000000000, 0.000000000000000000 ) ) ;
#1636=CARTESIAN_POINT ( 'NONE',  ( 47.00000000000000000, 1.133017633246824530E-14, 20.99999999999999645 ) ) ;
#1639=VECTOR ( 'NONE', #1876, 1000.000000000000000 ) ;
#1640=AXIS2_PLACEMENT_3D ( 'NONE', #99, #72, #574 ) ;
#1641=AXIS2_PLACEMENT_3D ( 'NONE', #1572, #1326, #2822 ) ;
#1645=CIRCLE ( 'NONE', #1481, 4.999999999999998224 ) ;
#1646=EDGE_LOOP ( 'NONE', ( #1389, #3044, #1676, #1069, #2280 ) ) ;
#1654=PRODUCT_DEFINITION_FORMATION_WITH_SPECIFIED_SOURCE ( 'ANY', '', #2716, .NOT_KNOWN. ) ;
#1660=FACE_BOUND ( 'NONE', #1725, .T. ) ;
#1662=ORIENTED_EDGE ( 'NONE', *, *, #2188, .T. ) ;
#1665=ORIENTED_EDGE ( 'NONE', *, *, #372, .F. ) ;
#1669=ORIENTED_EDGE ( 'NONE', *, *, #1088, .T. ) ;
#1673=ORIENTED_EDGE ( 'NONE', *, *, #1793, .F. ) ;
#1675=ADVANCED_FACE ( 'NONE', ( #1660, #3162 ), #2669, .F. ) ;
#1676=ORIENTED_EDGE ( 'NONE', *, *, #1172, .T. ) ;
#1678=VERTEX_POINT ( 'NONE', #1880 ) ;
#1679=CARTESIAN_POINT ( 'NONE',  ( 35.50000000000000711, 1.492884656567496302E-14, 20.99999999999999645 ) ) ;
#1685=CIRCLE ( 'NONE', #3025, 14.00000000000000000 ) ;
#1689=LINE ( 'NONE', #1249, #702 ) ;
#1693=CARTESIAN_POINT ( 'NONE',  ( 52.00000000000000711, 3.708099243547853252, 20.99999999999999645 ) ) ;
#1699=FACE_BOUND ( 'NONE', #1467, .T. ) ;
#1707=FACE_OUTER_BOUND ( 'NONE', #2787, .T. ) ;
#1708=CARTESIAN_POINT ( 'NONE',  ( 47.00000000000000000, -3.708099243547826607, 20.99999999999999645 ) ) ;
#1709=VERTEX_POINT ( 'NONE', #2175 ) ;
#1712=FACE_OUTER_BOUND ( 'NONE', #2856, .T. ) ;
#1714=CARTESIAN_POINT ( 'NONE',  ( 30.00000000000000000, 3.673940397442057600E-15, 15.00000000000000000 ) ) ;
#1715=LINE ( 'NONE', #1906, #1233 ) ;
#1725=EDGE_LOOP ( 'NONE', ( #3097, #1280 ) ) ;
#1726=DIRECTION ( 'NONE',  ( 1.000000000000000000, 2.312964634635742957E-16, -0.000000000000000000 ) ) ;
#1729=CARTESIAN_POINT ( 'NONE',  ( -41.99999999999999289, -15.00000000000000711, 0.000000000000000000 ) ) ;
#1741=DIRECTION ( 'NONE',  ( 1.000000000000000000, 2.312964634635742957E-16, -0.000000000000000000 ) ) ;
#1742=DIRECTION ( 'NONE',  ( 1.000000000000000000, -0.000000000000000000, -0.000000000000000000 ) ) ;
#1743=AXIS2_PLACEMENT_3D ( 'NONE', #1875, #837, #1097 ) ;
#1744=DIRECTION ( 'NONE',  ( -0.000000000000000000, -0.000000000000000000, 1.000000000000000000 ) ) ;
#1747=CIRCLE ( 'NONE', #66, 30.00000000000000000 ) ;
#1753=EDGE_CURVE ( 'NONE', #1678, #87, #3126, .T. ) ;
#1755=ORIENTED_EDGE ( 'NONE', *, *, #657, .T. ) ;
#1757=ADVANCED_FACE ( 'NONE', ( #2503 ), #960, .F. ) ;
#1762=FACE_OUTER_BOUND ( 'NONE', #2830, .T. ) ;
#1764=VECTOR ( 'NONE', #167, 1000.000000000000000 ) ;
#1766=DIRECTION ( 'NONE',  ( 1.000000000000000000, 2.312964634635742957E-16, 0.000000000000000000 ) ) ;
#1768=DIRECTION ( 'NONE',  ( -1.000000000000000000, 0.000000000000000000, 0.000000000000000000 ) ) ;
#1769=CARTESIAN_POINT ( 'NONE',  ( -37.00000000000000000, -5.785761963836251101E-15, 2.500000000000001332 ) ) ;
#1770=ORIENTED_EDGE ( 'NONE', *, *, #2879, .T. ) ;
#1774=CARTESIAN_POINT ( 'NONE',  ( 37.66466167501431528, -1.348281052163420091, 16.39851580165996836 ) ) ;
#1777=CARTESIAN_POINT ( 'NONE',  ( 35.50000000000000711, 1.492884656567496302E-14, 20.99999999999999645 ) ) ;
#1778=DIRECTION ( 'NONE',  ( 0.000000000000000000, -1.000000000000000000, 0.000000000000000000 ) ) ;
#1779=VERTEX_POINT ( 'NONE', #736 ) ;
#1781=CARTESIAN_POINT ( 'NONE',  ( 38.34772064623945909, 0.6658172387807621551, 16.47579882838004650 ) ) ;
#1784=AXIS2_PLACEMENT_3D ( 'NONE', #1714, #1741, #434 ) ;
#1785=ORIENTED_EDGE ( 'NONE', *, *, #2945, .T. ) ;
#1787=CARTESIAN_POINT ( 'NONE',  ( 35.50000000000000000, 1.243235838461289750E-14, 16.49999999999999289 ) ) ;
#1789=VERTEX_POINT ( 'NONE', #279 ) ;
#1792=AXIS2_PLACEMENT_3D ( 'NONE', #1, #1511, #1560 ) ;
#1793=EDGE_CURVE ( 'NONE', #1489, #2004, #1007, .T. ) ;
#1795=EDGE_LOOP ( 'NONE', ( #2032, #1358, #1497, #1411, #2892 ) ) ;
#1796=VECTOR ( 'NONE', #1348, 1000.000000000000000 ) ;
#1798=CARTESIAN_POINT ( 'NONE',  ( 35.65194399346782461, 0.6651260505907339304, 16.47584948644689007 ) ) ;
#1799=CARTESIAN_POINT ( 'NONE',  ( 47.00000000000000000, 1.133017633246824530E-14, 7.500000000000000000 ) ) ;
#1806=DIRECTION ( 'NONE',  ( 0.000000000000000000, 1.000000000000000000, 0.000000000000000000 ) ) ;
#1814=VECTOR ( 'NONE', #1923, 1000.000000000000000 ) ;
#1821=EDGE_CURVE ( 'NONE', #576, #974, #1405, .T. ) ;
#1824=CARTESIAN_POINT ( 'NONE',  ( 35.69898883018239388, 0.7529305858385579864, 16.46882038169668050 ) ) ;
#1825=AXIS2_PLACEMENT_3D ( 'NONE', #2933, #2996, #3194 ) ;
#1828=MECHANICAL_DESIGN_GEOMETRIC_PRESENTATION_REPRESENTATION('',(#1410),#801);
#1829=VERTEX_POINT ( 'NONE', #1769 ) ;
#1830=DIRECTION ( 'NONE',  ( -1.000000000000000000, -2.312964634635742957E-16, 0.000000000000000000 ) ) ;
#1837=DIRECTION ( 'NONE',  ( 1.000000000000000000, 0.000000000000000000, 0.000000000000000000 ) ) ;
#1839=CIRCLE ( 'NONE', #172, 8.999999999999994671 ) ;
#1842=ORIENTED_EDGE ( 'NONE', *, *, #147, .T. ) ;
#1843=CIRCLE ( 'NONE', #121, 14.00000000000000000 ) ;
#1846=DIRECTION ( 'NONE',  ( 1.000000000000000000, -0.000000000000000000, -0.000000000000000000 ) ) ;
#1847=CARTESIAN_POINT ( 'NONE',  ( 38.30993956269965395, -0.7564481093111403709, 16.46997477067511539 ) ) ;
#1853=LINE ( 'NONE', #2629, #1132 ) ;
#1857=LINE ( 'NONE', #2356, #2296 ) ;
#1859=CYLINDRICAL_SURFACE ( 'NONE', #900, 41.99999999999999289 ) ;
#1862=ORIENTED_EDGE ( 'NONE', *, *, #2720, .T. ) ;
#1867=PLANE ( 'NONE',  #1950 ) ;
#1875=CARTESIAN_POINT ( 'NONE',  ( 3.469446951953614189E-15, -15.00000000000000355, 15.00000000000000000 ) ) ;
#1876=DIRECTION ( 'NONE',  ( -0.000000000000000000, -0.000000000000000000, -1.000000000000000000 ) ) ;
#1877=VERTEX_POINT ( 'NONE', #973 ) ;
#1879=UNCERTAINTY_MEASURE_WITH_UNIT (LENGTH_MEASURE( 1.000000000000000082E-05 ), #776, 'distance_accuracy_value', 'NONE');
#1880=CARTESIAN_POINT ( 'NONE',  ( 41.99999999999999289, -13.99999999999999112, 7.500000000000001776 ) ) ;
#1882=VERTEX_POINT ( 'NONE', #1708 ) ;
#1889=ORIENTED_EDGE ( 'NONE', *, *, #2322, .T. ) ;
#1896=CARTESIAN_POINT ( 'NONE',  ( -41.99999999999999289, -15.00000000000000711, 15.00000000000000000 ) ) ;
#1899=STYLED_ITEM ( 'NONE', ( #1036 ), #1050 ) ;
#1900=CIRCLE ( 'NONE', #390, 4.999999999999999112 ) ;
#1906=CARTESIAN_POINT ( 'NONE',  ( 41.99999999999999289, 6.449497959004948951E-15, 0.000000000000000000 ) ) ;
#1908=ORIENTED_EDGE ( 'NONE', *, *, #2164, .T. ) ;
#1909=CARTESIAN_POINT ( 'NONE',  ( 27.00000000000000000, 1.133017633246824530E-14, 7.500000000000000000 ) ) ;
#1913=DIRECTION ( 'NONE',  ( 2.312964634635742957E-16, -1.000000000000000000, 0.000000000000000000 ) ) ;
#1918=ORIENTED_EDGE ( 'NONE', *, *, #1821, .T. ) ;
#1922=CARTESIAN_POINT ( 'NONE',  ( 27.00000000000000000, -3.708099243547831048, 20.99999999999999645 ) ) ;
#1923=DIRECTION ( 'NONE',  ( 1.000000000000000000, -0.000000000000000000, -0.000000000000000000 ) ) ;
#1928=DIRECTION ( 'NONE',  ( -1.000000000000000000, -2.312964634635743450E-16, -0.000000000000000000 ) ) ;
#1929=ORIENTED_EDGE ( 'NONE', *, *, #2879, .F. ) ;
#1934=ORIENTED_EDGE ( 'NONE', *, *, #2782, .F. ) ;
#1947=CIRCLE ( 'NONE', #2102, 7.500000000000000000 ) ;
#1948=ADVANCED_FACE ( 'NONE', ( #313 ), #297, .T. ) ;
#1950=AXIS2_PLACEMENT_3D ( 'NONE', #2066, #2851, #629 ) ;
#1953=DIRECTION ( 'NONE',  ( 0.000000000000000000, 0.000000000000000000, 1.000000000000000000 ) ) ;
#1958=DIRECTION ( 'NONE',  ( 0.000000000000000000, 0.000000000000000000, -1.000000000000000000 ) ) ;
#1964=VERTEX_POINT ( 'NONE', #1379 ) ;
#1967=FACE_OUTER_BOUND ( 'NONE', #232, .T. ) ;
#1977=ORIENTED_EDGE ( 'NONE', *, *, #893, .F. ) ;
#1978=ORIENTED_EDGE ( 'NONE', *, *, #943, .T. ) ;
#1995=CARTESIAN_POINT ( 'NONE',  ( 47.00000000000000000, 1.133017633246824530E-14, 7.500000000000000000 ) ) ;
#1996=CARTESIAN_POINT ( 'NONE',  ( 37.19571985532142833, -1.490394421081172371, 16.37575894629745932 ) ) ;
#1997=CARTESIAN_POINT ( 'NONE',  ( 47.00000000000000000, 1.133017633246824530E-14, -1.499999999999989120 ) ) ;
#2002=VECTOR ( 'NONE', #1195, 1000.000000000000000 ) ;
#2004=VERTEX_POINT ( 'NONE', #2767 ) ;
#2008=DIRECTION ( 'NONE',  ( 1.000000000000000000, 0.000000000000000000, 0.000000000000000000 ) ) ;
#2014=CARTESIAN_POINT ( 'NONE',  ( 30.00000000000000000, 7.398136453587482028E-15, 7.500000000000000000 ) ) ;
#2016=DIRECTION ( 'NONE',  ( 1.000000000000000000, 2.312964634635742957E-16, 0.000000000000000000 ) ) ;
#2017=UNCERTAINTY_MEASURE_WITH_UNIT (LENGTH_MEASURE( 1.000000000000000082E-05 ), #605, 'distance_accuracy_value', 'NONE');
#2018=DIRECTION ( 'NONE',  ( 1.000000000000000000, -0.000000000000000000, -0.000000000000000000 ) ) ;
#2019=ORIENTED_EDGE ( 'NONE', *, *, #2921, .F. ) ;
#2022=CARTESIAN_POINT ( 'NONE',  ( 38.49023808469348751, 0.1968962347057520990, 16.49835841594091335 ) ) ;
#2023=FILL_AREA_STYLE ('',( #826 ) ) ;
#2024=DIRECTION ( 'NONE',  ( 2.312964634635742957E-16, -1.000000000000000000, 0.000000000000000000 ) ) ;
#2028=ADVANCED_FACE ( 'NONE', ( #871 ), #2375, .F. ) ;
#2032=ORIENTED_EDGE ( 'NONE', *, *, #525, .T. ) ;
#2033=EDGE_CURVE ( 'NONE', #1503, #1789, #2524, .T. ) ;
#2038=CARTESIAN_POINT ( 'NONE',  ( 37.75516277711826518, 1.310683246666518365, 16.40437238582925872 ) ) ;
#2043=ORIENTED_EDGE ( 'NONE', *, *, #2828, .T. ) ;
#2045=CARTESIAN_POINT ( 'NONE',  ( 37.75078578997759848, -1.302282315510294941, 16.40545230064624249 ) ) ;
#2050=CARTESIAN_POINT ( 'NONE',  ( 27.00000000000000355, -13.99999999999999289, 7.500000000000001776 ) ) ;
#2053=ORIENTED_EDGE ( 'NONE', *, *, #2322, .F. ) ;
#2055=CARTESIAN_POINT ( 'NONE',  ( 36.61043004145793134, 1.451850406891378675, 16.38214551140935882 ) ) ;
#2060=ORIENTED_EDGE ( 'NONE', *, *, #1080, .F. ) ;
#2062=EDGE_CURVE ( 'NONE', #1393, #1599, #1857, .T. ) ;
#2066=CARTESIAN_POINT ( 'NONE',  ( 41.99999999999999289, 6.449497959004948951E-15, 15.00000000000000000 ) ) ;
#2067=CARTESIAN_POINT ( 'NONE',  ( 27.00000000000000355, -11.82159041753688200, 0.000000000000000000 ) ) ;
#2074=EDGE_LOOP ( 'NONE', ( #2, #1106, #2963, #1141 ) ) ;
#2078=APPLICATION_CONTEXT ( 'automotive_design' ) ;
#2081=CARTESIAN_POINT ( 'NONE',  ( 41.99999999999999289, -15.00000000000000355, 15.00000000000000000 ) ) ;
#2084=EDGE_CURVE ( 'NONE', #585, #1570, #530, .T. ) ;
#2086=ADVANCED_FACE ( 'NONE', ( #698 ), #206, .F. ) ;
#2089=CIRCLE ( 'NONE', #2600, 14.00000000000000000 ) ;
#2092=VERTEX_POINT ( 'NONE', #2170 ) ;
#2097=ORIENTED_EDGE ( 'NONE', *, *, #943, .F. ) ;
#2102=AXIS2_PLACEMENT_3D ( 'NONE', #3030, #3051, #2549 ) ;
#2106=LINE ( 'NONE', #1896, #1639 ) ;
#2124=AXIS2_PLACEMENT_3D ( 'NONE', #1260, #2018, #3006 ) ;
#2126=ORIENTED_EDGE ( 'NONE', *, *, #559, .F. ) ;
#2128=ORIENTED_EDGE ( 'NONE', *, *, #372, .T. ) ;
#2131=DIRECTION ( 'NONE',  ( 1.000000000000000000, 2.312964634635742957E-16, 0.000000000000000000 ) ) ;
#2136=MANIFOLD_SOLID_BREP ( 'Cut-Extrude-Thin1', #443 ) ;
#2146=DIRECTION ( 'NONE',  ( -1.000000000000000000, -2.312964634635742957E-16, 0.000000000000000000 ) ) ;
#2147=EDGE_CURVE ( 'NONE', #1134, #163, #650, .T. ) ;
#2152=CARTESIAN_POINT ( 'NONE',  ( -37.00000000000000000, -5.785761963836251101E-15, 7.500000000000000000 ) ) ;
#2159=VECTOR ( 'NONE', #2309, 1000.000000000000000 ) ;
#2161=VECTOR ( 'NONE', #710, 1000.000000000000000 ) ;
#2162=VECTOR ( 'NONE', #1928, 1000.000000000000000 ) ;
#2164=EDGE_CURVE ( 'NONE', #1964, #2636, #3004, .T. ) ;
#2165=DIRECTION ( 'NONE',  ( -1.000000000000000000, -2.312964634635742957E-16, 0.000000000000000000 ) ) ;
#2167=LINE ( 'NONE', #1165, #410 ) ;
#2170=CARTESIAN_POINT ( 'NONE',  ( 30.00000000000000000, -11.82159041753688200, 0.000000000000000000 ) ) ;
#2174=ORIENTED_EDGE ( 'NONE', *, *, #2945, .F. ) ;
#2175=CARTESIAN_POINT ( 'NONE',  ( -37.00000000000000000, -5.173438564262574571E-15, 12.49999999999999645 ) ) ;
#2183=LINE ( 'NONE', #1440, #1814 ) ;
#2185=EDGE_CURVE ( 'NONE', #1365, #3117, #289, .T. ) ;
#2188=EDGE_CURVE ( 'NONE', #779, #1561, #282, .T. ) ;
#2198=DIRECTION ( 'NONE',  ( 1.000000000000000000, 0.000000000000000000, -0.000000000000000000 ) ) ;
#2201=DIRECTION ( 'NONE',  ( 2.312964634635742957E-16, -1.000000000000000000, 0.000000000000000000 ) ) ;
#2213=AXIS2_PLACEMENT_3D ( 'NONE', #1277, #1494, #1294 ) ;
#2214=CIRCLE ( 'NONE', #2938, 1.499999999999994449 ) ;
#2216=CARTESIAN_POINT ( 'NONE',  ( 3.469446951953614189E-15, -15.00000000000000355, 0.000000000000000000 ) ) ;
#2223=DIRECTION ( 'NONE',  ( 1.000000000000000000, 0.000000000000000000, -0.000000000000000000 ) ) ;
#2239=LINE ( 'NONE', #2441, #116 ) ;
#2241=ORIENTED_EDGE ( 'NONE', *, *, #2759, .T. ) ;
#2242=ORIENTED_EDGE ( 'NONE', *, *, #1286, .F. ) ;
#2247=DIRECTION ( 'NONE',  ( 1.000000000000000000, 2.312964634635742957E-16, 0.000000000000000000 ) ) ;
#2248=EDGE_CURVE ( 'NONE', #1561, #779, #1900, .T. ) ;
#2251=ORIENTED_EDGE ( 'NONE', *, *, #147, .F. ) ;
#2252=DIRECTION ( 'NONE',  ( -1.000000000000000000, -2.312964634635742957E-16, 0.000000000000000000 ) ) ;
#2253=CARTESIAN_POINT ( 'NONE',  ( 52.00000000000000711, -3.708099243547825274, 20.99999999999999645 ) ) ;
#2259=CARTESIAN_POINT ( 'NONE',  ( 37.09819064725438409, -1.500059831078487171, 16.37410956135322948 ) ) ;
#2261=CIRCLE ( 'NONE', #2459, 8.999999999999989342 ) ;
#2269=FACE_OUTER_BOUND ( 'NONE', #1629, .T. ) ;
#2273=B_SPLINE_CURVE_WITH_KNOTS ( 'NONE', 3,
 ( #1787, #2773, #2806, #553, #2493, #73, #1041, #1542, #3002, #992, #1255, #2259, #1996, #2510, #16, #1774, #2045, #2757, #533, #287, #1847, #107, #366, #1351 ),
 .UNSPECIFIED., .F., .F.,
 ( 4, 2, 2, 2, 2, 2, 2, 2, 2, 2, 2, 4 ),
 ( 0.004697885398315485364, 0.005284974574641448583, 0.005872063750967410935, 0.006165608339130399483, 0.006459152927293387164, 0.007046242103619364261, 0.007339786691782353677, 0.007633331279945342225, 0.007926875868108331641, 0.008220420456271318455, 0.008807509632597297286, 0.009394598808923274383 ),
 .UNSPECIFIED. ) ;
#2280=ORIENTED_EDGE ( 'NONE', *, *, #772, .F. ) ;
#2283=CARTESIAN_POINT ( 'NONE',  ( 36.24410157368015462, 1.310477515366009760, 16.40440676504734085 ) ) ;
#2284=FACE_OUTER_BOUND ( 'NONE', #1293, .T. ) ;
#2295=CARTESIAN_POINT ( 'NONE',  ( 27.00000000000000000, 1.133017633246824688E-14, -1.499999999999994449 ) ) ;
#2296=VECTOR ( 'NONE', #393, 1000.000000000000000 ) ;
#2300=CARTESIAN_POINT ( 'NONE',  ( -41.99999999999999289, -6.449497959004950529E-15, 0.000000000000000000 ) ) ;
#2301=ORIENTED_EDGE ( 'NONE', *, *, #2921, .T. ) ;
#2303=ORIENTED_EDGE ( 'NONE', *, *, #3182, .T. ) ;
#2304=DIRECTION ( 'NONE',  ( 2.312964634635742957E-16, -1.000000000000000000, 0.000000000000000000 ) ) ;
#2307=ORIENTED_EDGE ( 'NONE', *, *, #931, .F. ) ;
#2309=DIRECTION ( 'NONE',  ( 1.000000000000000000, -0.000000000000000000, -0.000000000000000000 ) ) ;
#2315=AXIS2_PLACEMENT_3D ( 'NONE', #1995, #532, #2726 ) ;
#2316=DIRECTION ( 'NONE',  ( 1.000000000000000000, -0.000000000000000000, -0.000000000000000000 ) ) ;
#2322=EDGE_CURVE ( 'NONE', #163, #1134, #1839, .T. ) ;
#2323=CARTESIAN_POINT ( 'NONE',  ( -30.00000000000000000, -3.673940397442059178E-15, 15.00000000000000000 ) ) ;
#2327=DIRECTION ( 'NONE',  ( 1.000000000000000000, 2.312964634635742957E-16, 0.000000000000000000 ) ) ;
#2328=FACE_OUTER_BOUND ( 'NONE', #2379, .T. ) ;
#2329=VECTOR ( 'NONE', #1295, 1000.000000000000000 ) ;
#2331=LINE ( 'NONE', #158, #2670 ) ;
#2339=ORIENTED_EDGE ( 'NONE', *, *, #559, .T. ) ;
#2340=EDGE_CURVE ( 'NONE', #1599, #1482, #3041, .T. ) ;
#2356=CARTESIAN_POINT ( 'NONE',  ( -26.99999999999999645, -7.500000000000007105, 7.500000000000000000 ) ) ;
#2362=CARTESIAN_POINT ( 'NONE',  ( 3.469446951953614189E-15, -15.00000000000000355, 15.00000000000000000 ) ) ;
#2363=ORIENTED_EDGE ( 'NONE', *, *, #2164, .F. ) ;
#2374=EDGE_LOOP ( 'NONE', ( #1862, #2866, #1072, #1548, #1058 ) ) ;
#2375=CYLINDRICAL_SURFACE ( 'NONE', #2596, 4.999999999999999112 ) ;
#2376=FACE_BOUND ( 'NONE', #2803, .T. ) ;
#2379=EDGE_LOOP ( 'NONE', ( #324, #1755, #1343, #1665, #529, #1012, #2242, #2620 ) ) ;
#2381=DIRECTION ( 'NONE',  ( 0.000000000000000000, 0.000000000000000000, -1.000000000000000000 ) ) ;
#2386=FACE_OUTER_BOUND ( 'NONE', #690, .T. ) ;
#2397=VERTEX_POINT ( 'NONE', #1110 ) ;
#2400=DIRECTION ( 'NONE',  ( 1.000000000000000000, -0.000000000000000000, -0.000000000000000000 ) ) ;
#2403=ORIENTED_EDGE ( 'NONE', *, *, #2248, .F. ) ;
#2411=CARTESIAN_POINT ( 'NONE',  ( -26.99999999999999645, 7.499999999999992006, 7.500000000000000888 ) ) ;
#2412=CIRCLE ( 'NONE', #341, 14.00000000000000000 ) ;
#2416=DIRECTION ( 'NONE',  ( -2.478176394252581634E-16, 1.000000000000000000, 0.000000000000000000 ) ) ;
#2418=EDGE_CURVE ( 'NONE', #1829, #1561, #1077, .T. ) ;
#2424=CARTESIAN_POINT ( 'NONE',  ( 3.469446951953614189E-15, -15.00000000000000355, 15.00000000000000000 ) ) ;
#2429=CIRCLE ( 'NONE', #1021, 41.99999999999999289 ) ;
#2430=VERTEX_POINT ( 'NONE', #1624 ) ;
#2433=CARTESIAN_POINT ( 'NONE',  ( 27.00000000000000000, 6.704247063196759979E-15, 7.500000000000000000 ) ) ;
#2436=DIRECTION ( 'NONE',  ( 0.000000000000000000, 0.000000000000000000, -1.000000000000000000 ) ) ;
#2441=CARTESIAN_POINT ( 'NONE',  ( 27.00000000000000000, 3.708099243547847479, 20.99999999999999645 ) ) ;
#2447=ORIENTED_EDGE ( 'NONE', *, *, #2185, .T. ) ;
#2450=CARTESIAN_POINT ( 'NONE',  ( 27.00000000000000000, 6.704247063196759979E-15, 7.500000000000000000 ) ) ;
#2451=DIRECTION ( 'NONE',  ( -0.000000000000000000, -0.000000000000000000, -1.000000000000000000 ) ) ;
#2459=AXIS2_PLACEMENT_3D ( 'NONE', #1201, #190, #1958 ) ;
#2460=ADVANCED_FACE ( 'NONE', ( #353 ), #1867, .T. ) ;
#2465=AXIS2_PLACEMENT_3D ( 'NONE', #2424, #2995, #1768 ) ;
#2469=SHAPE_DEFINITION_REPRESENTATION ( #907, #514 ) ;
#2474=DIRECTION ( 'NONE',  ( -0.000000000000000000, -0.000000000000000000, 1.000000000000000000 ) ) ;
#2484=DIRECTION ( 'NONE',  ( 2.312964634635742957E-16, -1.000000000000000000, 0.000000000000000000 ) ) ;
#2488=CARTESIAN_POINT ( 'NONE',  ( 38.49999999999999289, 1.474514954580286030E-14, 20.99999999999999645 ) ) ;
#2493=CARTESIAN_POINT ( 'NONE',  ( 35.80050950286611311, -0.9216565616594013521, 16.45376772233409213 ) ) ;
#2494=CARTESIAN_POINT ( 'NONE',  ( 47.00000000000000000, 1.133017633246824530E-14, 7.500000000000000000 ) ) ;
#2503=FACE_OUTER_BOUND ( 'NONE', #1795, .T. ) ;
#2507=AXIS2_PLACEMENT_3D ( 'NONE', #538, #308, #2484 ) ;
#2510=CARTESIAN_POINT ( 'NONE',  ( 37.38775466693719807, -1.452318184980603721, 16.38206869443958169 ) ) ;
#2521=MECHANICAL_DESIGN_GEOMETRIC_PRESENTATION_REPRESENTATION('',(#1899),#3089);
#2523=CARTESIAN_POINT ( 'NONE',  ( 36.07902659818448399, 1.200345445641991970, 16.42070378373879080 ) ) ;
#2524=LINE ( 'NONE', #2300, #2919 ) ;
#2526=ORIENTED_EDGE ( 'NONE', *, *, #575, .F. ) ;
#2529=CARTESIAN_POINT ( 'NONE',  ( 30.00000000000000000, 7.398136453587482028E-15, 7.500000000000000000 ) ) ;
#2531=ORIENTED_EDGE ( 'NONE', *, *, #2147, .F. ) ;
#2534=CARTESIAN_POINT ( 'NONE',  ( 36.90254329834230873, 1.500037116461215625, 16.37411340082286770 ) ) ;
#2536=EDGE_CURVE ( 'NONE', #56, #1829, #2925, .T. ) ;
#2544=CARTESIAN_POINT ( 'NONE',  ( 27.00000000000000000, 3.708099243547847479, 20.99999999999999645 ) ) ;
#2549=DIRECTION ( 'NONE',  ( 0.000000000000000000, -1.000000000000000000, 0.000000000000000000 ) ) ;
#2551=ORIENTED_EDGE ( 'NONE', *, *, #1793, .T. ) ;
#2552=ADVANCED_FACE ( 'NONE', ( #1712 ), #2893, .T. ) ;
#2560=DIRECTION ( 'NONE',  ( -2.312964634635742957E-16, 1.000000000000000000, -0.000000000000000000 ) ) ;
#2561=ORIENTED_EDGE ( 'NONE', *, *, #713, .F. ) ;
#2567=ORIENTED_EDGE ( 'NONE', *, *, #3166, .T. ) ;
#2576=ORIENTED_EDGE ( 'NONE', *, *, #1753, .T. ) ;
#2580=AXIS2_PLACEMENT_3D ( 'NONE', #2494, #2987, #1806 ) ;
#2583=LINE ( 'NONE', #593, #392 ) ;
#2587=DIRECTION ( 'NONE',  ( 1.000000000000000000, 2.312964634635742957E-16, 0.000000000000000000 ) ) ;
#2589=ORIENTED_EDGE ( 'NONE', *, *, #2062, .F. ) ;
#2596=AXIS2_PLACEMENT_3D ( 'NONE', #782, #1534, #118 ) ;
#2600=AXIS2_PLACEMENT_3D ( 'NONE', #1469, #1726, #727 ) ;
#2603=EDGE_LOOP ( 'NONE', ( #1929, #2905, #3039 ) ) ;
#2607=ORIENTED_EDGE ( 'NONE', *, *, #598, .F. ) ;
#2616=VECTOR ( 'NONE', #2304, 1000.000000000000000 ) ;
#2618=CARTESIAN_POINT ( 'NONE',  ( 47.00000000000000000, 1.133017633246824530E-14, 7.500000000000000000 ) ) ;
#2620=ORIENTED_EDGE ( 'NONE', *, *, #2828, .F. ) ;
#2625=DIRECTION ( 'NONE',  ( 1.000000000000000000, 0.000000000000000000, 0.000000000000000000 ) ) ;
#2628=ADVANCED_FACE ( 'NONE', ( #2386 ), #148, .T. ) ;
#2629=CARTESIAN_POINT ( 'NONE',  ( 47.00000000000000000, 1.133017633246824530E-14, -1.499999999999994449 ) ) ;
#2631=ORIENTED_EDGE ( 'NONE', *, *, #51, .F. ) ;
#2636=VERTEX_POINT ( 'NONE', #1679 ) ;
#2642=ORIENTED_EDGE ( 'NONE', *, *, #7, .F. ) ;
#2651=AXIS2_PLACEMENT_3D ( 'NONE', #1236, #750, #511 ) ;
#2656=EDGE_CURVE ( 'NONE', #357, #1678, #2089, .T. ) ;
#2663=CARTESIAN_POINT ( 'NONE',  ( 41.99999999999999289, -15.00000000000000355, 0.000000000000000000 ) ) ;
#2669=PLANE ( 'NONE',  #1602 ) ;
#2670=VECTOR ( 'NONE', #1913, 1000.000000000000000 ) ;
#2671=VECTOR ( 'NONE', #2941, 1000.000000000000000 ) ;
#2673=CARTESIAN_POINT ( 'NONE',  ( 30.00000000000000355, -13.99999999999999467, 7.500000000000001776 ) ) ;
#2675=CIRCLE ( 'NONE', #1271, 7.500000000000000000 ) ;
#2680=PLANE ( 'NONE',  #102 ) ;
#2684=ADVANCED_FACE ( 'NONE', ( #729 ), #2708, .F. ) ;
#2691=VECTOR ( 'NONE', #835, 1000.000000000000000 ) ;
#2705=ORIENTED_EDGE ( 'NONE', *, *, #931, .T. ) ;
#2708=PLANE ( 'NONE',  #790 ) ;
#2710=B_SPLINE_CURVE_WITH_KNOTS ( 'NONE', 3,
 ( #327, #2751, #2022, #3061, #2783, #1781, #71, #1549, #1248, #526, #2038, #1314, #2798, #2534, #1071, #2055, #1532, #2283, #2523, #1002, #825, #1824, #1798, #3026, #796, #508, #54, #561 ),
 .UNSPECIFIED., .F., .F.,
 ( 4, 2, 2, 2, 2, 2, 2, 2, 2, 2, 2, 2, 2, 4 ),
 ( 0.000000000000000000, 0.0002936178373947212505, 0.0005872356747894425010, 0.0008808535121841636973, 0.001174471349578885002, 0.001761707024368327828, 0.002348942699157770871, 0.002642560536552492501, 0.002936178373947213264, 0.003523414048736636574, 0.003817031886131348663, 0.004110649723526061186, 0.004404267560920773275, 0.004697885398315485364 ),
 .UNSPECIFIED. ) ;
#2713=VERTEX_POINT ( 'NONE', #682 ) ;
#2716=PRODUCT ( 'frame', 'frame', '', ( #485 ) ) ;
#2718=CIRCLE ( 'NONE', #1792, 7.500000000000000000 ) ;
#2720=EDGE_CURVE ( 'NONE', #916, #3031, #1229, .T. ) ;
#2726=DIRECTION ( 'NONE',  ( 0.000000000000000000, 1.000000000000000000, 0.000000000000000000 ) ) ;
#2730=ADVANCED_FACE ( 'NONE', ( #741 ), #3150, .F. ) ;
#2736=ADVANCED_FACE ( 'NONE', ( #1967 ), #3185, .F. ) ;
#2737=LINE ( 'NONE', #2253, #2162 ) ;
#2739=VERTEX_POINT ( 'NONE', #1922 ) ;
#2741=APPLICATION_CONTEXT ( 'automotive_design' ) ;
#2744=AXIS2_PLACEMENT_3D ( 'NONE', #1133, #2131, #3113 ) ;
#2745=DIRECTION ( 'NONE',  ( 1.000000000000000000, 2.312964634635742957E-16, -0.000000000000000000 ) ) ;
#2750=ORIENTED_EDGE ( 'NONE', *, *, #1192, .T. ) ;
#2751=CARTESIAN_POINT ( 'NONE',  ( 38.49999999999999289, 0.09929498707318666628, 16.49999999999999289 ) ) ;
#2752=CARTESIAN_POINT ( 'NONE',  ( 37.00000000000000000, 1.474514954580286030E-14, 20.99999999999999645 ) ) ;
#2755=ORIENTED_EDGE ( 'NONE', *, *, #2084, .T. ) ;
#2757=CARTESIAN_POINT ( 'NONE',  ( 37.91396272957889124, -1.193436492094909429, 16.42069107455876775 ) ) ;
#2759=EDGE_CURVE ( 'NONE', #2739, #1365, #1685, .T. ) ;
#2767=CARTESIAN_POINT ( 'NONE',  ( 38.49999999999999289, 1.474514954580286030E-14, 20.99999999999999645 ) ) ;
#2770=AXIS2_PLACEMENT_3D ( 'NONE', #1360, #120, #1631 ) ;
#2772=DIRECTION ( 'NONE',  ( 0.000000000000000000, 0.000000000000000000, -1.000000000000000000 ) ) ;
#2773=CARTESIAN_POINT ( 'NONE',  ( 35.50000000000000000, -0.1959257125632785645, 16.49999999999999289 ) ) ;
#2777=DIRECTION ( 'NONE',  ( -3.854941057726240069E-16, 1.000000000000000000, 0.000000000000000000 ) ) ;
#2780=CARTESIAN_POINT ( 'NONE',  ( -41.99999999999999289, -6.449497959004950529E-15, 15.00000000000000000 ) ) ;
#2782=EDGE_CURVE ( 'NONE', #2965, #974, #2926, .T. ) ;
#2783=CARTESIAN_POINT ( 'NONE',  ( 38.42308964188128328, 0.4842307372812582611, 16.48742442505516692 ) ) ;
#2787=EDGE_LOOP ( 'NONE', ( #2097, #962, #1785, #3013, #1567, #2908, #1538, #2631 ) ) ;
#2797=ADVANCED_FACE ( 'NONE', ( #1699, #1471 ), #2680, .F. ) ;
#2798=CARTESIAN_POINT ( 'NONE',  ( 37.19662223785018540, 1.499925442620323235, 16.37413227714582220 ) ) ;
#2799=DIRECTION ( 'NONE',  ( 0.000000000000000000, 0.000000000000000000, 1.000000000000000000 ) ) ;
#2803=EDGE_LOOP ( 'NONE', ( #2307, #2817 ) ) ;
#2806=CARTESIAN_POINT ( 'NONE',  ( 35.53942839536624376, -0.3936020622859607854, 16.49320894598177034 ) ) ;
#2812=EDGE_LOOP ( 'NONE', ( #2251, #1056, #2128, #2750 ) ) ;
#2815=SHAPE_REPRESENTATION_RELATIONSHIP ( 'NONE' , 'NONE' ,  #514, #1050 ) ;
#2817=ORIENTED_EDGE ( 'NONE', *, *, #2084, .F. ) ;
#2821=VERTEX_POINT ( 'NONE', #33 ) ;
#2822=DIRECTION ( 'NONE',  ( 0.000000000000000000, -1.000000000000000000, 0.000000000000000000 ) ) ;
#2828=EDGE_CURVE ( 'NONE', #3117, #2092, #1627, .T. ) ;
#2830=EDGE_LOOP ( 'NONE', ( #2561, #2126 ) ) ;
#2851=DIRECTION ( 'NONE',  ( 1.000000000000000000, 2.312964634635742957E-16, -0.000000000000000000 ) ) ;
#2856=EDGE_LOOP ( 'NONE', ( #2863, #2339, #1225, #2060, #299, #2642 ) ) ;
#2863=ORIENTED_EDGE ( 'NONE', *, *, #273, .F. ) ;
#2866=ORIENTED_EDGE ( 'NONE', *, *, #1092, .T. ) ;
#2867=CARTESIAN_POINT ( 'NONE',  ( -41.99999999999999289, -1.109217911451089172E-14, 15.00000000000000000 ) ) ;
#2868=EDGE_LOOP ( 'NONE', ( #1977, #2301, #2043, #802, #367 ) ) ;
#2878=AXIS2_PLACEMENT_3D ( 'NONE', #3071, #2799, #1837 ) ;
#2879=EDGE_CURVE ( 'NONE', #56, #1709, #818, .T. ) ;
#2887=CARTESIAN_POINT ( 'NONE',  ( 27.00000000000000355, -13.99999999999999289, 7.500000000000001776 ) ) ;
#2892=ORIENTED_EDGE ( 'NONE', *, *, #2782, .T. ) ;
#2893=CYLINDRICAL_SURFACE ( 'NONE', #654, 7.500000000000000000 ) ;
#2894=DIRECTION ( 'NONE',  ( 2.312964634635742957E-16, -1.000000000000000000, 0.000000000000000000 ) ) ;
#2901=DIRECTION ( 'NONE',  ( 1.000000000000000000, -0.000000000000000000, -0.000000000000000000 ) ) ;
#2905=ORIENTED_EDGE ( 'NONE', *, *, #2536, .T. ) ;
#2908=ORIENTED_EDGE ( 'NONE', *, *, #2720, .F. ) ;
#2910=DIRECTION ( 'NONE',  ( 1.000000000000000000, 2.312964634635742957E-16, 0.000000000000000000 ) ) ;
#2919=VECTOR ( 'NONE', #1359, 1000.000000000000000 ) ;
#2921=EDGE_CURVE ( 'NONE', #2713, #3117, #1843, .T. ) ;
#2924=EDGE_CURVE ( 'NONE', #1964, #1489, #2273, .T. ) ;
#2925=LINE ( 'NONE', #693, #2671 ) ;
#2926=LINE ( 'NONE', #695, #3184 ) ;
#2927=CARTESIAN_POINT ( 'NONE',  ( -26.99999999999999645, -7.500000000000007105, 7.500000000000000000 ) ) ;
#2933=CARTESIAN_POINT ( 'NONE',  ( -30.00000000000000000, -3.673940397442059178E-15, 15.00000000000000000 ) ) ;
#2938=AXIS2_PLACEMENT_3D ( 'NONE', #2752, #1005, #2008 ) ;
#2941=DIRECTION ( 'NONE',  ( 0.5150380749100542666, 0.000000000000000000, -0.8571673007021122226 ) ) ;
#2945=EDGE_CURVE ( 'NONE', #2821, #2965, #1747, .T. ) ;
#2951=AXIS2_PLACEMENT_3D ( 'NONE', #883, #2587, #1068 ) ;
#2957=CARTESIAN_POINT ( 'NONE',  ( 38.49999999999999289, 1.474514954580286030E-14, 16.49999999999999289 ) ) ;
#2958=DIRECTION ( 'NONE',  ( 1.000000000000000000, -0.000000000000000000, -0.000000000000000000 ) ) ;
#2963=ORIENTED_EDGE ( 'NONE', *, *, #839, .T. ) ;
#2965=VERTEX_POINT ( 'NONE', #846 ) ;
#2968=CARTESIAN_POINT ( 'NONE',  ( -41.99999999999999289, -6.449497959004950529E-15, 15.00000000000000000 ) ) ;
#2975=DIRECTION ( 'NONE',  ( 0.000000000000000000, 0.000000000000000000, 1.000000000000000000 ) ) ;
#2987=DIRECTION ( 'NONE',  ( 1.000000000000000000, 2.312964634635742957E-16, 0.000000000000000000 ) ) ;
#2990=CARTESIAN_POINT ( 'NONE',  ( 37.00000000000000000, 1.474514954580286030E-14, 20.99999999999999645 ) ) ;
#2995=DIRECTION ( 'NONE',  ( -0.000000000000000000, -0.000000000000000000, -1.000000000000000000 ) ) ;
#2996=DIRECTION ( 'NONE',  ( -1.000000000000000000, -2.312964634635742957E-16, 0.000000000000000000 ) ) ;
#2998=VERTEX_POINT ( 'NONE', #335 ) ;
#3001=VECTOR ( 'NONE', #631, 1000.000000000000000 ) ;
#3002=CARTESIAN_POINT ( 'NONE',  ( 36.33339417452629050, -1.347339434735542074, 16.39865934157270644 ) ) ;
#3004=LINE ( 'NONE', #1777, #1105 ) ;
#3006=DIRECTION ( 'NONE',  ( 0.000000000000000000, 0.000000000000000000, -1.000000000000000000 ) ) ;
#3010=CYLINDRICAL_SURFACE ( 'NONE', #1640, 1.499999999999994449 ) ;
#3011=CARTESIAN_POINT ( 'NONE',  ( -41.99999999999999289, -6.449497959004950529E-15, 15.00000000000000000 ) ) ;
#3013=ORIENTED_EDGE ( 'NONE', *, *, #1303, .T. ) ;
#3015=LINE ( 'NONE', #1087, #2616 ) ;
#3017=CARTESIAN_POINT ( 'NONE',  ( -26.99999999999999645, -5.785761963836251101E-15, 2.500000000000000444 ) ) ;
#3020=CARTESIAN_POINT ( 'NONE',  ( -26.99999999999999645, -5.785761963836251101E-15, 7.500000000000000000 ) ) ;
#3024=ORIENTED_EDGE ( 'NONE', *, *, #2656, .T. ) ;
#3025=AXIS2_PLACEMENT_3D ( 'NONE', #2433, #2910, #3169 ) ;
#3026=CARTESIAN_POINT ( 'NONE',  ( 35.57671993710908964, 0.4836543419624541595, 16.48745487577124180 ) ) ;
#3027=( NAMED_UNIT ( * ) SI_UNIT ( $, .STERADIAN. ) SOLID_ANGLE_UNIT ( ) );
#3030=CARTESIAN_POINT ( 'NONE',  ( -41.99999999999999289, -1.109217911451089172E-14, 7.500000000000000000 ) ) ;
#3031=VERTEX_POINT ( 'NONE', #2867 ) ;
#3032=CIRCLE ( 'NONE', #1743, 41.99999999999999289 ) ;
#3039=ORIENTED_EDGE ( 'NONE', *, *, #598, .T. ) ;
#3040=( NAMED_UNIT ( * ) SI_UNIT ( $, .STERADIAN. ) SOLID_ANGLE_UNIT ( ) );
#3041=CIRCLE ( 'NONE', #1641, 7.500000000000000000 ) ;
#3044=ORIENTED_EDGE ( 'NONE', *, *, #51, .T. ) ;
#3051=DIRECTION ( 'NONE',  ( -1.000000000000000000, -2.312964634635742957E-16, 0.000000000000000000 ) ) ;
#3053=DIRECTION ( 'NONE',  ( -2.478176394252581634E-16, 1.000000000000000000, 0.000000000000000000 ) ) ;
#3057=LINE ( 'NONE', #2081, #3001 ) ;
#3058=ORIENTED_EDGE ( 'NONE', *, *, #1490, .F. ) ;
#3059=VECTOR ( 'NONE', #2560, 1000.000000000000000 ) ;
#3061=CARTESIAN_POINT ( 'NONE',  ( 38.45202114561161011, 0.3888602178275711863, 16.49210820886665019 ) ) ;
#3062=ORIENTED_EDGE ( 'NONE', *, *, #2147, .T. ) ;
#3063=CARTESIAN_POINT ( 'NONE',  ( 27.00000000000000000, 6.704247063196759979E-15, 7.500000000000000000 ) ) ;
#3071=CARTESIAN_POINT ( 'NONE',  ( 0.000000000000000000, 0.000000000000000000, 0.000000000000000000 ) ) ;
#3074=EDGE_LOOP ( 'NONE', ( #1842, #2303, #1237, #129 ) ) ;
#3076=CARTESIAN_POINT ( 'NONE',  ( -37.00000000000000000, -5.785761963836251101E-15, 7.500000000000000000 ) ) ;
#3079=CIRCLE ( 'NONE', #1258, 1.499999999999994449 ) ;
#3089=( GEOMETRIC_REPRESENTATION_CONTEXT ( 3 ) GLOBAL_UNCERTAINTY_ASSIGNED_CONTEXT ( ( #777 ) ) GLOBAL_UNIT_ASSIGNED_CONTEXT ( ( #1533, #1082, #3027 ) ) REPRESENTATION_CONTEXT ( 'NONE', 'WORKASPACE' ) );
#3097=ORIENTED_EDGE ( 'NONE', *, *, #1067, .F. ) ;
#3105=DIRECTION ( 'NONE',  ( -1.000000000000000000, 0.000000000000000000, 0.000000000000000000 ) ) ;
#3111=ORIENTED_EDGE ( 'NONE', *, *, #273, .T. ) ;
#3113=DIRECTION ( 'NONE',  ( -2.478176394252581634E-16, 1.000000000000000000, 0.000000000000000000 ) ) ;
#3116=ORIENTED_EDGE ( 'NONE', *, *, #2033, .T. ) ;
#3117=VERTEX_POINT ( 'NONE', #2673 ) ;
#3126=LINE ( 'NONE', #2887, #869 ) ;
#3127=AXIS2_PLACEMENT_3D ( 'NONE', #918, #2400, #217 ) ;
#3128=VERTEX_POINT ( 'NONE', #2411 ) ;
#3131=DIRECTION ( 'NONE',  ( 0.000000000000000000, -1.000000000000000000, 0.000000000000000000 ) ) ;
#3134=ORIENTED_EDGE ( 'NONE', *, *, #1508, .T. ) ;
#3141=VECTOR ( 'NONE', #1254, 1000.000000000000000 ) ;
#3143=ORIENTED_EDGE ( 'NONE', *, *, #1092, .F. ) ;
#3146=EDGE_LOOP ( 'NONE', ( #382, #3134, #1662, #1033 ) ) ;
#3147=CARTESIAN_POINT ( 'NONE',  ( 47.00000000000000000, 1.243235845170086321E-14, 16.49999999999999289 ) ) ;
#3150=PLANE ( 'NONE',  #1784 ) ;
#3155=LINE ( 'NONE', #924, #746 ) ;
#3157=ADVANCED_FACE ( 'NONE', ( #2269 ), #198, .F. ) ;
#3162=FACE_OUTER_BOUND ( 'NONE', #3074, .T. ) ;
#3166=EDGE_CURVE ( 'NONE', #1489, #585, #1401, .T. ) ;
#3169=DIRECTION ( 'NONE',  ( -2.478176394252581634E-16, 1.000000000000000000, 0.000000000000000000 ) ) ;
#3173=DIRECTION ( 'NONE',  ( 0.000000000000000000, -1.000000000000000000, 0.000000000000000000 ) ) ;
#3181=ORIENTED_EDGE ( 'NONE', *, *, #2188, .F. ) ;
#3182=EDGE_CURVE ( 'NONE', #2430, #1128, #1436, .T. ) ;
#3184=VECTOR ( 'NONE', #469, 1000.000000000000000 ) ;
#3185=CYLINDRICAL_SURFACE ( 'NONE', #3127, 4.999999999999999112 ) ;
#3194=DIRECTION ( 'NONE',  ( 2.312964634635742957E-16, -1.000000000000000000, 0.000000000000000000 ) ) ;
#3195=ORIENTED_EDGE ( 'NONE', *, *, #397, .T. ) ;
#3198=ADVANCED_FACE ( 'NONE', ( #1052 ), #450, .F. ) ;
#3204=CARTESIAN_POINT ( 'NONE',  ( 27.00000000000000000, 6.704247063196759979E-15, 7.500000000000000000 ) ) ;
#3211=ADVANCED_FACE ( 'NONE', ( #2284 ), #3010, .F. ) ;
#3216=DIRECTION ( 'NONE',  ( -2.312964634635742957E-16, 1.000000000000000000, 0.000000000000000000 ) ) ;
#3219=ADVANCED_FACE ( 'NONE', ( #2328 ), #346, .T. ) ;
#3230=COLOUR_RGB('Dark Blue',0.08,0.2,0.34);
#3231=FILL_AREA_STYLE_COLOUR('',#3230);
#3232=FILL_AREA_STYLE('',(#3231));
#3233=SURFACE_STYLE_FILL_AREA(#3232);
#3234=SURFACE_SIDE_STYLE('',(#3233));
#3235=SURFACE_STYLE_USAGE(.BOTH.,#3234);
#3236=PRESENTATION_STYLE_ASSIGNMENT((#3235));
ENDSEC;
END-ISO-10303-21;
